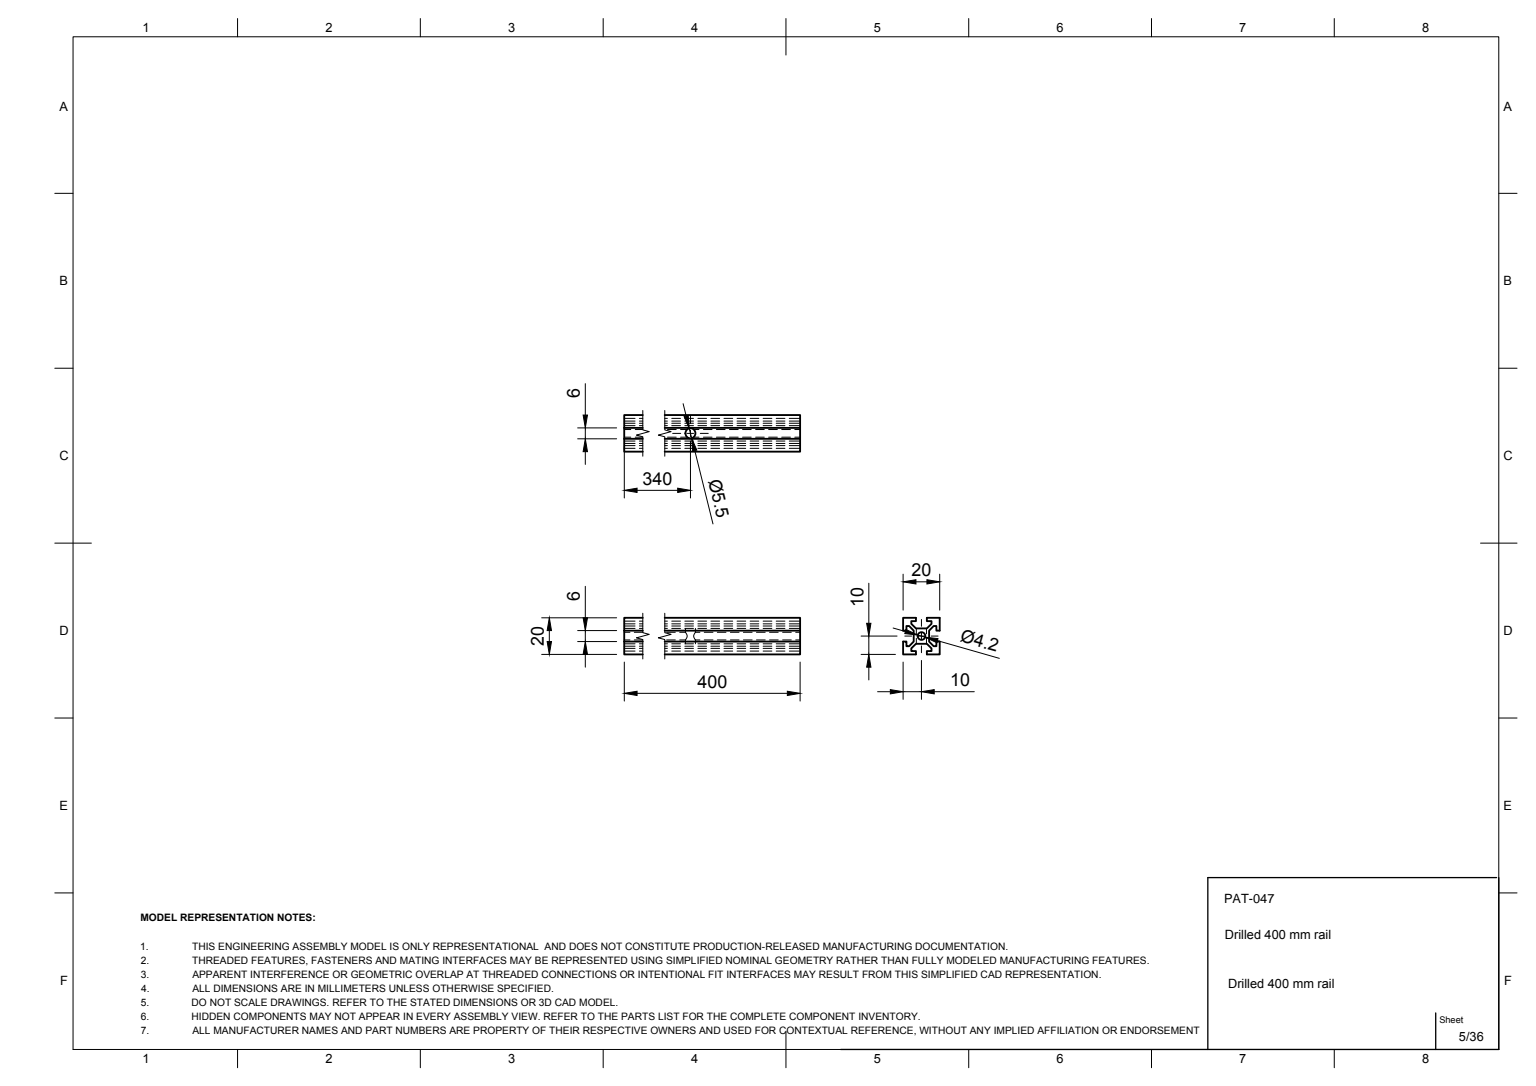
ISO-10303-21;
HEADER;
/* Generated by software containing ST-Developer
 * from STEP Tools, Inc. (www.steptools.com) 
 */

FILE_DESCRIPTION(
/* description */ ('Gravity roller conveyor section'),
/* implementation_level */ '2;1');

FILE_NAME(
/* name */ 'Drilled 400 mm rail.step',
/* time_stamp */ '2026-11-02T07:43:02-08:00',
/* author */ (''),
/* organization */ (''),
/* preprocessor_version */ 'ST-DEVELOPER v20.2',
/* originating_system */ 'Autodesk Translation Framework v15.17.0.0',
/* authorisation */ '');

FILE_SCHEMA (('AUTOMOTIVE_DESIGN { 1 0 10303 214 3 1 1 }'));
ENDSEC;

DATA;
#10=MECHANICAL_DESIGN_GEOMETRIC_PRESENTATION_REPRESENTATION('',(#530),#13821);
#433=B_SPLINE_CURVE_WITH_KNOTS('',3,(#11133,#11134,#11135,#11136,#11137,
#11138,#11139,#11140,#11141,#11142,#11143,#11144,#11145,#11146,#11147,#11148,
#11149,#11150,#11151,#11152,#11153,#11154),.UNSPECIFIED.,.F.,.F.,(4,2,2,
2,2,2,2,2,2,2,4),(0.335938049981194,0.418928967949028,0.501919885916861,
0.586897992939625,0.629387046451007,0.671876099962389,0.714365153473771,
0.756854206985153,0.841832314007917,0.92482323197575,1.00781414994358),
 .UNSPECIFIED.);
#434=B_SPLINE_CURVE_WITH_KNOTS('',3,(#11159,#11160,#11161,#11162,#11163,
#11164,#11165,#11166,#11167,#11168,#11169,#11170),.UNSPECIFIED.,.F.,.F.,
(4,2,2,2,2,4),(0.,0.0424890535113821,0.0849781070227642,0.169956214045528,
0.252947132013361,0.335938049981194),.UNSPECIFIED.);
#435=B_SPLINE_CURVE_WITH_KNOTS('',3,(#11171,#11172,#11173,#11174,#11175,
#11176,#11177,#11178,#11179,#11180,#11181,#11182),.UNSPECIFIED.,.F.,.F.,
(4,2,2,2,2,4),(1.00781414994358,1.09080506791142,1.17379598587925,1.25877409290201,
1.3012631464134,1.34375219992478),.UNSPECIFIED.);
#436=B_SPLINE_CURVE_WITH_KNOTS('',3,(#11185,#11186,#11187,#11188,#11189,
#11190,#11191,#11192,#11193,#11194,#11195,#11196,#11197,#11198,#11199,#11200,
#11201,#11202,#11203,#11204,#11205,#11206,#11207,#11208,#11209,#11210,#11211,
#11212,#11213,#11214,#11215,#11216),.UNSPECIFIED.,.F.,.F.,(4,2,2,2,2,2,
2,2,2,2,2,2,2,2,2,4),(0.,0.0424890535113822,0.0849781070227643,0.169956214045529,
0.252947132013362,0.335938049981195,0.418928967949028,0.501919885916861,
0.586897992939625,0.629387046451007,0.671876099962389,0.714365153473771,
0.756854206985153,0.841832314007917,0.924823231975751,1.00781414994358),
 .UNSPECIFIED.);
#437=B_SPLINE_CURVE_WITH_KNOTS('',3,(#11217,#11218,#11219,#11220,#11221,
#11222,#11223,#11224,#11225,#11226,#11227,#11228),.UNSPECIFIED.,.F.,.F.,
(4,2,2,2,2,4),(1.00781414994358,1.09080506791142,1.17379598587925,1.25877409290201,
1.3012631464134,1.34375219992478),.UNSPECIFIED.);
#462=SHAPE_REPRESENTATION_RELATIONSHIP('SRR','None',#13999,#496);
#496=ADVANCED_BREP_SHAPE_REPRESENTATION('',(#572),#13786);
#530=STYLED_ITEM('',(#14191),#572);
#572=MANIFOLD_SOLID_BREP('Body1',#7628);
#617=FACE_BOUND('',#1445,.T.);
#618=FACE_BOUND('',#1461,.T.);
#619=FACE_BOUND('',#1480,.T.);
#620=FACE_BOUND('',#1495,.T.);
#621=FACE_BOUND('',#1497,.T.);
#708=PLANE('',#8075);
#709=PLANE('',#8076);
#710=PLANE('',#8077);
#711=PLANE('',#8078);
#712=PLANE('',#8079);
#713=PLANE('',#8080);
#714=PLANE('',#8081);
#715=PLANE('',#8082);
#716=PLANE('',#8083);
#717=PLANE('',#8084);
#718=PLANE('',#8085);
#719=PLANE('',#8086);
#720=PLANE('',#8087);
#721=PLANE('',#8088);
#722=PLANE('',#8089);
#723=PLANE('',#8090);
#724=PLANE('',#8091);
#725=PLANE('',#8092);
#726=PLANE('',#8093);
#727=PLANE('',#8094);
#728=PLANE('',#8095);
#729=PLANE('',#8096);
#730=PLANE('',#8097);
#731=PLANE('',#8098);
#732=PLANE('',#8099);
#733=PLANE('',#8100);
#734=PLANE('',#8101);
#735=PLANE('',#8102);
#736=PLANE('',#8103);
#737=PLANE('',#8104);
#738=PLANE('',#8105);
#739=PLANE('',#8106);
#740=PLANE('',#8107);
#741=PLANE('',#8108);
#742=PLANE('',#8109);
#743=PLANE('',#8110);
#744=PLANE('',#8113);
#745=PLANE('',#8114);
#746=PLANE('',#8115);
#747=PLANE('',#8116);
#748=PLANE('',#8117);
#749=PLANE('',#8118);
#750=PLANE('',#8119);
#751=PLANE('',#8120);
#752=PLANE('',#8121);
#753=PLANE('',#8122);
#1017=FACE_OUTER_BOUND('',#1444,.T.);
#1018=FACE_OUTER_BOUND('',#1446,.T.);
#1019=FACE_OUTER_BOUND('',#1447,.T.);
#1020=FACE_OUTER_BOUND('',#1448,.T.);
#1021=FACE_OUTER_BOUND('',#1449,.T.);
#1022=FACE_OUTER_BOUND('',#1450,.T.);
#1023=FACE_OUTER_BOUND('',#1451,.T.);
#1024=FACE_OUTER_BOUND('',#1452,.T.);
#1025=FACE_OUTER_BOUND('',#1453,.T.);
#1026=FACE_OUTER_BOUND('',#1454,.T.);
#1027=FACE_OUTER_BOUND('',#1455,.T.);
#1028=FACE_OUTER_BOUND('',#1456,.T.);
#1029=FACE_OUTER_BOUND('',#1457,.T.);
#1030=FACE_OUTER_BOUND('',#1458,.T.);
#1031=FACE_OUTER_BOUND('',#1459,.T.);
#1032=FACE_OUTER_BOUND('',#1460,.T.);
#1033=FACE_OUTER_BOUND('',#1462,.T.);
#1034=FACE_OUTER_BOUND('',#1463,.T.);
#1035=FACE_OUTER_BOUND('',#1464,.T.);
#1036=FACE_OUTER_BOUND('',#1465,.T.);
#1037=FACE_OUTER_BOUND('',#1466,.T.);
#1038=FACE_OUTER_BOUND('',#1467,.T.);
#1039=FACE_OUTER_BOUND('',#1468,.T.);
#1040=FACE_OUTER_BOUND('',#1469,.T.);
#1041=FACE_OUTER_BOUND('',#1470,.T.);
#1042=FACE_OUTER_BOUND('',#1471,.T.);
#1043=FACE_OUTER_BOUND('',#1472,.T.);
#1044=FACE_OUTER_BOUND('',#1473,.T.);
#1045=FACE_OUTER_BOUND('',#1474,.T.);
#1046=FACE_OUTER_BOUND('',#1475,.T.);
#1047=FACE_OUTER_BOUND('',#1476,.T.);
#1048=FACE_OUTER_BOUND('',#1477,.T.);
#1049=FACE_OUTER_BOUND('',#1478,.T.);
#1050=FACE_OUTER_BOUND('',#1479,.T.);
#1051=FACE_OUTER_BOUND('',#1481,.T.);
#1052=FACE_OUTER_BOUND('',#1482,.T.);
#1053=FACE_OUTER_BOUND('',#1483,.T.);
#1054=FACE_OUTER_BOUND('',#1484,.T.);
#1055=FACE_OUTER_BOUND('',#1485,.T.);
#1056=FACE_OUTER_BOUND('',#1486,.T.);
#1057=FACE_OUTER_BOUND('',#1487,.T.);
#1058=FACE_OUTER_BOUND('',#1488,.T.);
#1059=FACE_OUTER_BOUND('',#1489,.T.);
#1060=FACE_OUTER_BOUND('',#1490,.T.);
#1061=FACE_OUTER_BOUND('',#1491,.T.);
#1062=FACE_OUTER_BOUND('',#1492,.T.);
#1063=FACE_OUTER_BOUND('',#1493,.T.);
#1064=FACE_OUTER_BOUND('',#1494,.T.);
#1065=FACE_OUTER_BOUND('',#1496,.T.);
#1444=EDGE_LOOP('',(#5250,#5251,#5252,#5253,#5254,#5255,#5256,#5257,#5258));
#1445=EDGE_LOOP('',(#5259,#5260));
#1446=EDGE_LOOP('',(#5261,#5262,#5263,#5264,#5265,#5266));
#1447=EDGE_LOOP('',(#5267,#5268,#5269,#5270));
#1448=EDGE_LOOP('',(#5271,#5272,#5273,#5274));
#1449=EDGE_LOOP('',(#5275,#5276,#5277,#5278));
#1450=EDGE_LOOP('',(#5279,#5280,#5281,#5282));
#1451=EDGE_LOOP('',(#5283,#5284,#5285,#5286));
#1452=EDGE_LOOP('',(#5287,#5288,#5289,#5290));
#1453=EDGE_LOOP('',(#5291,#5292,#5293,#5294));
#1454=EDGE_LOOP('',(#5295,#5296,#5297,#5298));
#1455=EDGE_LOOP('',(#5299,#5300,#5301,#5302));
#1456=EDGE_LOOP('',(#5303,#5304,#5305,#5306));
#1457=EDGE_LOOP('',(#5307,#5308,#5309,#5310));
#1458=EDGE_LOOP('',(#5311,#5312,#5313,#5314));
#1459=EDGE_LOOP('',(#5315,#5316,#5317,#5318));
#1460=EDGE_LOOP('',(#5319,#5320,#5321,#5322));
#1461=EDGE_LOOP('',(#5323));
#1462=EDGE_LOOP('',(#5324,#5325,#5326,#5327));
#1463=EDGE_LOOP('',(#5328,#5329,#5330,#5331));
#1464=EDGE_LOOP('',(#5332,#5333,#5334,#5335));
#1465=EDGE_LOOP('',(#5336,#5337,#5338,#5339));
#1466=EDGE_LOOP('',(#5340,#5341,#5342,#5343));
#1467=EDGE_LOOP('',(#5344,#5345,#5346,#5347));
#1468=EDGE_LOOP('',(#5348,#5349,#5350,#5351));
#1469=EDGE_LOOP('',(#5352,#5353,#5354,#5355));
#1470=EDGE_LOOP('',(#5356,#5357,#5358,#5359));
#1471=EDGE_LOOP('',(#5360,#5361,#5362,#5363));
#1472=EDGE_LOOP('',(#5364,#5365,#5366,#5367));
#1473=EDGE_LOOP('',(#5368,#5369,#5370,#5371));
#1474=EDGE_LOOP('',(#5372,#5373,#5374,#5375));
#1475=EDGE_LOOP('',(#5376,#5377,#5378,#5379));
#1476=EDGE_LOOP('',(#5380,#5381,#5382,#5383));
#1477=EDGE_LOOP('',(#5384,#5385,#5386,#5387));
#1478=EDGE_LOOP('',(#5388,#5389,#5390,#5391));
#1479=EDGE_LOOP('',(#5392,#5393,#5394,#5395));
#1480=EDGE_LOOP('',(#5396));
#1481=EDGE_LOOP('',(#5397,#5398,#5399,#5400));
#1482=EDGE_LOOP('',(#5401,#5402,#5403,#5404));
#1483=EDGE_LOOP('',(#5405,#5406,#5407,#5408));
#1484=EDGE_LOOP('',(#5409,#5410,#5411,#5412));
#1485=EDGE_LOOP('',(#5413,#5414,#5415,#5416,#5417));
#1486=EDGE_LOOP('',(#5418,#5419,#5420,#5421));
#1487=EDGE_LOOP('',(#5422,#5423,#5424,#5425));
#1488=EDGE_LOOP('',(#5426,#5427,#5428,#5429));
#1489=EDGE_LOOP('',(#5430,#5431,#5432,#5433));
#1490=EDGE_LOOP('',(#5434,#5435,#5436,#5437));
#1491=EDGE_LOOP('',(#5438,#5439,#5440,#5441));
#1492=EDGE_LOOP('',(#5442,#5443,#5444,#5445));
#1493=EDGE_LOOP('',(#5446,#5447,#5448,#5449));
#1494=EDGE_LOOP('',(#5450,#5451,#5452,#5453,#5454,#5455,#5456,#5457,#5458,
#5459,#5460,#5461,#5462,#5463,#5464,#5465,#5466,#5467,#5468,#5469,#5470,
#5471,#5472,#5473,#5474,#5475,#5476,#5477,#5478,#5479,#5480,#5481,#5482,
#5483,#5484,#5485,#5486,#5487,#5488,#5489,#5490,#5491,#5492,#5493));
#1495=EDGE_LOOP('',(#5494));
#1496=EDGE_LOOP('',(#5495,#5496,#5497,#5498,#5499,#5500,#5501,#5502,#5503,
#5504,#5505,#5506,#5507,#5508,#5509,#5510,#5511,#5512,#5513,#5514,#5515,
#5516,#5517,#5518,#5519,#5520,#5521,#5522,#5523,#5524,#5525,#5526,#5527,
#5528,#5529,#5530,#5531,#5532,#5533,#5534,#5535,#5536,#5537,#5538));
#1497=EDGE_LOOP('',(#5539));
#1954=LINE('',#11131,#2672);
#1955=LINE('',#11156,#2673);
#1956=LINE('',#11232,#2674);
#1957=LINE('',#11236,#2675);
#1958=LINE('',#11238,#2676);
#1959=LINE('',#11240,#2677);
#1960=LINE('',#11241,#2678);
#1961=LINE('',#11244,#2679);
#1962=LINE('',#11246,#2680);
#1963=LINE('',#11247,#2681);
#1964=LINE('',#11250,#2682);
#1965=LINE('',#11252,#2683);
#1966=LINE('',#11253,#2684);
#1967=LINE('',#11256,#2685);
#1968=LINE('',#11258,#2686);
#1969=LINE('',#11259,#2687);
#1970=LINE('',#11262,#2688);
#1971=LINE('',#11264,#2689);
#1972=LINE('',#11265,#2690);
#1973=LINE('',#11268,#2691);
#1974=LINE('',#11270,#2692);
#1975=LINE('',#11271,#2693);
#1976=LINE('',#11274,#2694);
#1977=LINE('',#11276,#2695);
#1978=LINE('',#11277,#2696);
#1979=LINE('',#11280,#2697);
#1980=LINE('',#11282,#2698);
#1981=LINE('',#11283,#2699);
#1982=LINE('',#11286,#2700);
#1983=LINE('',#11288,#2701);
#1984=LINE('',#11289,#2702);
#1985=LINE('',#11293,#2703);
#1986=LINE('',#11295,#2704);
#1987=LINE('',#11297,#2705);
#1988=LINE('',#11298,#2706);
#1989=LINE('',#11301,#2707);
#1990=LINE('',#11303,#2708);
#1991=LINE('',#11304,#2709);
#1992=LINE('',#11307,#2710);
#1993=LINE('',#11309,#2711);
#1994=LINE('',#11310,#2712);
#1995=LINE('',#11313,#2713);
#1996=LINE('',#11315,#2714);
#1997=LINE('',#11316,#2715);
#1998=LINE('',#11319,#2716);
#1999=LINE('',#11321,#2717);
#2000=LINE('',#11322,#2718);
#2001=LINE('',#11325,#2719);
#2002=LINE('',#11327,#2720);
#2003=LINE('',#11328,#2721);
#2004=LINE('',#11331,#2722);
#2005=LINE('',#11333,#2723);
#2006=LINE('',#11334,#2724);
#2007=LINE('',#11337,#2725);
#2008=LINE('',#11339,#2726);
#2009=LINE('',#11340,#2727);
#2010=LINE('',#11343,#2728);
#2011=LINE('',#11345,#2729);
#2012=LINE('',#11346,#2730);
#2013=LINE('',#11350,#2731);
#2014=LINE('',#11352,#2732);
#2015=LINE('',#11354,#2733);
#2016=LINE('',#11355,#2734);
#2017=LINE('',#11358,#2735);
#2018=LINE('',#11360,#2736);
#2019=LINE('',#11361,#2737);
#2020=LINE('',#11364,#2738);
#2021=LINE('',#11366,#2739);
#2022=LINE('',#11367,#2740);
#2023=LINE('',#11370,#2741);
#2024=LINE('',#11372,#2742);
#2025=LINE('',#11373,#2743);
#2026=LINE('',#11376,#2744);
#2027=LINE('',#11378,#2745);
#2028=LINE('',#11379,#2746);
#2029=LINE('',#11382,#2747);
#2030=LINE('',#11384,#2748);
#2031=LINE('',#11385,#2749);
#2032=LINE('',#11388,#2750);
#2033=LINE('',#11390,#2751);
#2034=LINE('',#11391,#2752);
#2035=LINE('',#11394,#2753);
#2036=LINE('',#11396,#2754);
#2037=LINE('',#11397,#2755);
#2038=LINE('',#11400,#2756);
#2039=LINE('',#11402,#2757);
#2040=LINE('',#11403,#2758);
#2041=LINE('',#11407,#2759);
#2042=LINE('',#11409,#2760);
#2043=LINE('',#11411,#2761);
#2044=LINE('',#11412,#2762);
#2045=LINE('',#11415,#2763);
#2046=LINE('',#11417,#2764);
#2047=LINE('',#11418,#2765);
#2048=LINE('',#11421,#2766);
#2049=LINE('',#11423,#2767);
#2050=LINE('',#11424,#2768);
#2051=LINE('',#11427,#2769);
#2052=LINE('',#11429,#2770);
#2053=LINE('',#11430,#2771);
#2054=LINE('',#11433,#2772);
#2055=LINE('',#11435,#2773);
#2056=LINE('',#11436,#2774);
#2057=LINE('',#11439,#2775);
#2058=LINE('',#11441,#2776);
#2059=LINE('',#11442,#2777);
#2060=LINE('',#11445,#2778);
#2061=LINE('',#11447,#2779);
#2062=LINE('',#11448,#2780);
#2063=LINE('',#11451,#2781);
#2064=LINE('',#11453,#2782);
#2065=LINE('',#11454,#2783);
#2066=LINE('',#11457,#2784);
#2067=LINE('',#11459,#2785);
#2068=LINE('',#11460,#2786);
#2069=LINE('',#11463,#2787);
#2070=LINE('',#11467,#2788);
#2071=LINE('',#11469,#2789);
#2072=LINE('',#11470,#2790);
#2073=LINE('',#11473,#2791);
#2074=LINE('',#11475,#2792);
#2075=LINE('',#11476,#2793);
#2076=LINE('',#11478,#2794);
#2077=LINE('',#11479,#2795);
#2078=LINE('',#11482,#2796);
#2079=LINE('',#11484,#2797);
#2080=LINE('',#11485,#2798);
#2081=LINE('',#11487,#2799);
#2082=LINE('',#11488,#2800);
#2083=LINE('',#11491,#2801);
#2084=LINE('',#11493,#2802);
#2085=LINE('',#11494,#2803);
#2086=LINE('',#11496,#2804);
#2087=LINE('',#11497,#2805);
#2088=LINE('',#11499,#2806);
#2089=LINE('',#11500,#2807);
#2672=VECTOR('',#8881,0.275);
#2673=VECTOR('',#8882,0.275);
#2674=VECTOR('',#8889,0.21);
#2675=VECTOR('',#8892,1.);
#2676=VECTOR('',#8893,1.);
#2677=VECTOR('',#8894,1.);
#2678=VECTOR('',#8895,1.);
#2679=VECTOR('',#8898,1.);
#2680=VECTOR('',#8899,1.);
#2681=VECTOR('',#8900,1.);
#2682=VECTOR('',#8903,1.);
#2683=VECTOR('',#8904,1.);
#2684=VECTOR('',#8905,1.);
#2685=VECTOR('',#8908,1.);
#2686=VECTOR('',#8909,1.);
#2687=VECTOR('',#8910,1.);
#2688=VECTOR('',#8913,1.);
#2689=VECTOR('',#8914,1.);
#2690=VECTOR('',#8915,1.);
#2691=VECTOR('',#8918,1.);
#2692=VECTOR('',#8919,1.);
#2693=VECTOR('',#8920,1.);
#2694=VECTOR('',#8923,1.);
#2695=VECTOR('',#8924,1.);
#2696=VECTOR('',#8925,1.);
#2697=VECTOR('',#8928,1.);
#2698=VECTOR('',#8929,1.);
#2699=VECTOR('',#8930,1.);
#2700=VECTOR('',#8933,1.);
#2701=VECTOR('',#8934,1.);
#2702=VECTOR('',#8935,1.);
#2703=VECTOR('',#8938,1.);
#2704=VECTOR('',#8939,1.);
#2705=VECTOR('',#8940,1.);
#2706=VECTOR('',#8941,1.);
#2707=VECTOR('',#8944,1.);
#2708=VECTOR('',#8945,1.);
#2709=VECTOR('',#8946,1.);
#2710=VECTOR('',#8949,1.);
#2711=VECTOR('',#8950,1.);
#2712=VECTOR('',#8951,1.);
#2713=VECTOR('',#8954,1.);
#2714=VECTOR('',#8955,1.);
#2715=VECTOR('',#8956,1.);
#2716=VECTOR('',#8959,1.);
#2717=VECTOR('',#8960,1.);
#2718=VECTOR('',#8961,1.);
#2719=VECTOR('',#8964,1.);
#2720=VECTOR('',#8965,1.);
#2721=VECTOR('',#8966,1.);
#2722=VECTOR('',#8969,1.);
#2723=VECTOR('',#8970,1.);
#2724=VECTOR('',#8971,1.);
#2725=VECTOR('',#8974,1.);
#2726=VECTOR('',#8975,1.);
#2727=VECTOR('',#8976,1.);
#2728=VECTOR('',#8979,1.);
#2729=VECTOR('',#8980,1.);
#2730=VECTOR('',#8981,1.);
#2731=VECTOR('',#8984,1.);
#2732=VECTOR('',#8985,1.);
#2733=VECTOR('',#8986,1.);
#2734=VECTOR('',#8987,1.);
#2735=VECTOR('',#8990,1.);
#2736=VECTOR('',#8991,1.);
#2737=VECTOR('',#8992,1.);
#2738=VECTOR('',#8995,1.);
#2739=VECTOR('',#8996,1.);
#2740=VECTOR('',#8997,1.);
#2741=VECTOR('',#9000,1.);
#2742=VECTOR('',#9001,1.);
#2743=VECTOR('',#9002,1.);
#2744=VECTOR('',#9005,1.);
#2745=VECTOR('',#9006,1.);
#2746=VECTOR('',#9007,1.);
#2747=VECTOR('',#9010,1.);
#2748=VECTOR('',#9011,1.);
#2749=VECTOR('',#9012,1.);
#2750=VECTOR('',#9015,1.);
#2751=VECTOR('',#9016,1.);
#2752=VECTOR('',#9017,1.);
#2753=VECTOR('',#9020,1.);
#2754=VECTOR('',#9021,1.);
#2755=VECTOR('',#9022,1.);
#2756=VECTOR('',#9025,1.);
#2757=VECTOR('',#9026,1.);
#2758=VECTOR('',#9027,1.);
#2759=VECTOR('',#9030,1.);
#2760=VECTOR('',#9031,1.);
#2761=VECTOR('',#9032,1.);
#2762=VECTOR('',#9033,1.);
#2763=VECTOR('',#9036,1.);
#2764=VECTOR('',#9037,1.);
#2765=VECTOR('',#9038,1.);
#2766=VECTOR('',#9041,1.);
#2767=VECTOR('',#9042,1.);
#2768=VECTOR('',#9043,1.);
#2769=VECTOR('',#9046,1.);
#2770=VECTOR('',#9047,1.);
#2771=VECTOR('',#9048,1.);
#2772=VECTOR('',#9051,1.);
#2773=VECTOR('',#9052,1.);
#2774=VECTOR('',#9053,1.);
#2775=VECTOR('',#9056,1.);
#2776=VECTOR('',#9057,1.);
#2777=VECTOR('',#9058,1.);
#2778=VECTOR('',#9061,1.);
#2779=VECTOR('',#9062,1.);
#2780=VECTOR('',#9063,1.);
#2781=VECTOR('',#9066,1.);
#2782=VECTOR('',#9067,1.);
#2783=VECTOR('',#9068,1.);
#2784=VECTOR('',#9071,1.);
#2785=VECTOR('',#9072,1.);
#2786=VECTOR('',#9073,1.);
#2787=VECTOR('',#9076,0.21);
#2788=VECTOR('',#9081,1.);
#2789=VECTOR('',#9082,1.);
#2790=VECTOR('',#9083,1.);
#2791=VECTOR('',#9086,1.);
#2792=VECTOR('',#9087,1.);
#2793=VECTOR('',#9088,1.);
#2794=VECTOR('',#9091,1.);
#2795=VECTOR('',#9092,1.);
#2796=VECTOR('',#9095,1.);
#2797=VECTOR('',#9096,1.);
#2798=VECTOR('',#9097,1.);
#2799=VECTOR('',#9100,1.);
#2800=VECTOR('',#9101,1.);
#2801=VECTOR('',#9104,1.);
#2802=VECTOR('',#9105,1.);
#2803=VECTOR('',#9106,1.);
#2804=VECTOR('',#9109,1.);
#2805=VECTOR('',#9110,1.);
#2806=VECTOR('',#9113,1.);
#2807=VECTOR('',#9114,1.);
#3382=CIRCLE('',#8071,0.275);
#3383=CIRCLE('',#8072,0.275);
#3384=CIRCLE('',#8074,0.21);
#3385=CIRCLE('',#8112,0.21);
#3606=VERTEX_POINT('',#11128);
#3607=VERTEX_POINT('',#11130);
#3608=VERTEX_POINT('',#11132);
#3609=VERTEX_POINT('',#11155);
#3610=VERTEX_POINT('',#11158);
#3611=VERTEX_POINT('',#11183);
#3612=VERTEX_POINT('',#11184);
#3613=VERTEX_POINT('',#11230);
#3614=VERTEX_POINT('',#11234);
#3615=VERTEX_POINT('',#11235);
#3616=VERTEX_POINT('',#11237);
#3617=VERTEX_POINT('',#11239);
#3618=VERTEX_POINT('',#11243);
#3619=VERTEX_POINT('',#11245);
#3620=VERTEX_POINT('',#11249);
#3621=VERTEX_POINT('',#11251);
#3622=VERTEX_POINT('',#11255);
#3623=VERTEX_POINT('',#11257);
#3624=VERTEX_POINT('',#11261);
#3625=VERTEX_POINT('',#11263);
#3626=VERTEX_POINT('',#11267);
#3627=VERTEX_POINT('',#11269);
#3628=VERTEX_POINT('',#11273);
#3629=VERTEX_POINT('',#11275);
#3630=VERTEX_POINT('',#11279);
#3631=VERTEX_POINT('',#11281);
#3632=VERTEX_POINT('',#11285);
#3633=VERTEX_POINT('',#11287);
#3634=VERTEX_POINT('',#11291);
#3635=VERTEX_POINT('',#11292);
#3636=VERTEX_POINT('',#11294);
#3637=VERTEX_POINT('',#11296);
#3638=VERTEX_POINT('',#11300);
#3639=VERTEX_POINT('',#11302);
#3640=VERTEX_POINT('',#11306);
#3641=VERTEX_POINT('',#11308);
#3642=VERTEX_POINT('',#11312);
#3643=VERTEX_POINT('',#11314);
#3644=VERTEX_POINT('',#11318);
#3645=VERTEX_POINT('',#11320);
#3646=VERTEX_POINT('',#11324);
#3647=VERTEX_POINT('',#11326);
#3648=VERTEX_POINT('',#11330);
#3649=VERTEX_POINT('',#11332);
#3650=VERTEX_POINT('',#11336);
#3651=VERTEX_POINT('',#11338);
#3652=VERTEX_POINT('',#11342);
#3653=VERTEX_POINT('',#11344);
#3654=VERTEX_POINT('',#11348);
#3655=VERTEX_POINT('',#11349);
#3656=VERTEX_POINT('',#11351);
#3657=VERTEX_POINT('',#11353);
#3658=VERTEX_POINT('',#11357);
#3659=VERTEX_POINT('',#11359);
#3660=VERTEX_POINT('',#11363);
#3661=VERTEX_POINT('',#11365);
#3662=VERTEX_POINT('',#11369);
#3663=VERTEX_POINT('',#11371);
#3664=VERTEX_POINT('',#11375);
#3665=VERTEX_POINT('',#11377);
#3666=VERTEX_POINT('',#11381);
#3667=VERTEX_POINT('',#11383);
#3668=VERTEX_POINT('',#11387);
#3669=VERTEX_POINT('',#11389);
#3670=VERTEX_POINT('',#11393);
#3671=VERTEX_POINT('',#11395);
#3672=VERTEX_POINT('',#11399);
#3673=VERTEX_POINT('',#11401);
#3674=VERTEX_POINT('',#11405);
#3675=VERTEX_POINT('',#11406);
#3676=VERTEX_POINT('',#11408);
#3677=VERTEX_POINT('',#11410);
#3678=VERTEX_POINT('',#11414);
#3679=VERTEX_POINT('',#11416);
#3680=VERTEX_POINT('',#11420);
#3681=VERTEX_POINT('',#11422);
#3682=VERTEX_POINT('',#11426);
#3683=VERTEX_POINT('',#11428);
#3684=VERTEX_POINT('',#11432);
#3685=VERTEX_POINT('',#11434);
#3686=VERTEX_POINT('',#11438);
#3687=VERTEX_POINT('',#11440);
#3688=VERTEX_POINT('',#11444);
#3689=VERTEX_POINT('',#11446);
#3690=VERTEX_POINT('',#11450);
#3691=VERTEX_POINT('',#11452);
#3692=VERTEX_POINT('',#11456);
#3693=VERTEX_POINT('',#11458);
#3694=VERTEX_POINT('',#11462);
#3695=VERTEX_POINT('',#11466);
#3696=VERTEX_POINT('',#11468);
#3697=VERTEX_POINT('',#11472);
#3698=VERTEX_POINT('',#11474);
#3699=VERTEX_POINT('',#11481);
#3700=VERTEX_POINT('',#11483);
#3701=VERTEX_POINT('',#11490);
#3702=VERTEX_POINT('',#11492);
#4262=EDGE_CURVE('',#3606,#3606,#3382,.T.);
#4263=EDGE_CURVE('',#3606,#3607,#1954,.T.);
#4264=EDGE_CURVE('',#3608,#3607,#433,.T.);
#4265=EDGE_CURVE('',#3608,#3609,#1955,.T.);
#4266=EDGE_CURVE('',#3609,#3609,#3383,.T.);
#4267=EDGE_CURVE('',#3610,#3608,#434,.T.);
#4268=EDGE_CURVE('',#3607,#3610,#435,.T.);
#4269=EDGE_CURVE('',#3611,#3612,#436,.T.);
#4270=EDGE_CURVE('',#3612,#3611,#437,.T.);
#4271=EDGE_CURVE('',#3613,#3613,#3384,.T.);
#4272=EDGE_CURVE('',#3613,#3608,#1956,.T.);
#4273=EDGE_CURVE('',#3614,#3615,#1957,.T.);
#4274=EDGE_CURVE('',#3614,#3616,#1958,.T.);
#4275=EDGE_CURVE('',#3617,#3616,#1959,.T.);
#4276=EDGE_CURVE('',#3615,#3617,#1960,.T.);
#4277=EDGE_CURVE('',#3618,#3614,#1961,.T.);
#4278=EDGE_CURVE('',#3618,#3619,#1962,.T.);
#4279=EDGE_CURVE('',#3616,#3619,#1963,.T.);
#4280=EDGE_CURVE('',#3620,#3618,#1964,.T.);
#4281=EDGE_CURVE('',#3620,#3621,#1965,.T.);
#4282=EDGE_CURVE('',#3619,#3621,#1966,.T.);
#4283=EDGE_CURVE('',#3622,#3620,#1967,.T.);
#4284=EDGE_CURVE('',#3622,#3623,#1968,.T.);
#4285=EDGE_CURVE('',#3621,#3623,#1969,.T.);
#4286=EDGE_CURVE('',#3624,#3622,#1970,.T.);
#4287=EDGE_CURVE('',#3624,#3625,#1971,.T.);
#4288=EDGE_CURVE('',#3623,#3625,#1972,.T.);
#4289=EDGE_CURVE('',#3626,#3624,#1973,.T.);
#4290=EDGE_CURVE('',#3626,#3627,#1974,.T.);
#4291=EDGE_CURVE('',#3625,#3627,#1975,.T.);
#4292=EDGE_CURVE('',#3628,#3626,#1976,.T.);
#4293=EDGE_CURVE('',#3628,#3629,#1977,.T.);
#4294=EDGE_CURVE('',#3627,#3629,#1978,.T.);
#4295=EDGE_CURVE('',#3630,#3628,#1979,.T.);
#4296=EDGE_CURVE('',#3630,#3631,#1980,.T.);
#4297=EDGE_CURVE('',#3629,#3631,#1981,.T.);
#4298=EDGE_CURVE('',#3632,#3630,#1982,.T.);
#4299=EDGE_CURVE('',#3633,#3632,#1983,.T.);
#4300=EDGE_CURVE('',#3631,#3633,#1984,.T.);
#4301=EDGE_CURVE('',#3634,#3635,#1985,.T.);
#4302=EDGE_CURVE('',#3634,#3636,#1986,.T.);
#4303=EDGE_CURVE('',#3637,#3636,#1987,.T.);
#4304=EDGE_CURVE('',#3635,#3637,#1988,.T.);
#4305=EDGE_CURVE('',#3638,#3634,#1989,.T.);
#4306=EDGE_CURVE('',#3638,#3639,#1990,.T.);
#4307=EDGE_CURVE('',#3636,#3639,#1991,.T.);
#4308=EDGE_CURVE('',#3640,#3638,#1992,.T.);
#4309=EDGE_CURVE('',#3640,#3641,#1993,.T.);
#4310=EDGE_CURVE('',#3639,#3641,#1994,.T.);
#4311=EDGE_CURVE('',#3642,#3640,#1995,.T.);
#4312=EDGE_CURVE('',#3642,#3643,#1996,.T.);
#4313=EDGE_CURVE('',#3641,#3643,#1997,.T.);
#4314=EDGE_CURVE('',#3644,#3642,#1998,.T.);
#4315=EDGE_CURVE('',#3644,#3645,#1999,.T.);
#4316=EDGE_CURVE('',#3643,#3645,#2000,.T.);
#4317=EDGE_CURVE('',#3646,#3644,#2001,.T.);
#4318=EDGE_CURVE('',#3646,#3647,#2002,.T.);
#4319=EDGE_CURVE('',#3645,#3647,#2003,.T.);
#4320=EDGE_CURVE('',#3648,#3646,#2004,.T.);
#4321=EDGE_CURVE('',#3648,#3649,#2005,.T.);
#4322=EDGE_CURVE('',#3647,#3649,#2006,.T.);
#4323=EDGE_CURVE('',#3650,#3648,#2007,.T.);
#4324=EDGE_CURVE('',#3650,#3651,#2008,.T.);
#4325=EDGE_CURVE('',#3649,#3651,#2009,.T.);
#4326=EDGE_CURVE('',#3652,#3650,#2010,.T.);
#4327=EDGE_CURVE('',#3653,#3652,#2011,.T.);
#4328=EDGE_CURVE('',#3651,#3653,#2012,.T.);
#4329=EDGE_CURVE('',#3654,#3655,#2013,.T.);
#4330=EDGE_CURVE('',#3654,#3656,#2014,.T.);
#4331=EDGE_CURVE('',#3657,#3656,#2015,.T.);
#4332=EDGE_CURVE('',#3655,#3657,#2016,.T.);
#4333=EDGE_CURVE('',#3658,#3654,#2017,.T.);
#4334=EDGE_CURVE('',#3658,#3659,#2018,.T.);
#4335=EDGE_CURVE('',#3656,#3659,#2019,.T.);
#4336=EDGE_CURVE('',#3660,#3658,#2020,.T.);
#4337=EDGE_CURVE('',#3660,#3661,#2021,.T.);
#4338=EDGE_CURVE('',#3659,#3661,#2022,.T.);
#4339=EDGE_CURVE('',#3662,#3660,#2023,.T.);
#4340=EDGE_CURVE('',#3662,#3663,#2024,.T.);
#4341=EDGE_CURVE('',#3661,#3663,#2025,.T.);
#4342=EDGE_CURVE('',#3664,#3662,#2026,.T.);
#4343=EDGE_CURVE('',#3664,#3665,#2027,.T.);
#4344=EDGE_CURVE('',#3663,#3665,#2028,.T.);
#4345=EDGE_CURVE('',#3666,#3664,#2029,.T.);
#4346=EDGE_CURVE('',#3666,#3667,#2030,.T.);
#4347=EDGE_CURVE('',#3665,#3667,#2031,.T.);
#4348=EDGE_CURVE('',#3668,#3666,#2032,.T.);
#4349=EDGE_CURVE('',#3668,#3669,#2033,.T.);
#4350=EDGE_CURVE('',#3667,#3669,#2034,.T.);
#4351=EDGE_CURVE('',#3670,#3668,#2035,.T.);
#4352=EDGE_CURVE('',#3670,#3671,#2036,.T.);
#4353=EDGE_CURVE('',#3669,#3671,#2037,.T.);
#4354=EDGE_CURVE('',#3672,#3670,#2038,.T.);
#4355=EDGE_CURVE('',#3673,#3672,#2039,.T.);
#4356=EDGE_CURVE('',#3671,#3673,#2040,.T.);
#4357=EDGE_CURVE('',#3674,#3675,#2041,.T.);
#4358=EDGE_CURVE('',#3674,#3676,#2042,.T.);
#4359=EDGE_CURVE('',#3677,#3676,#2043,.T.);
#4360=EDGE_CURVE('',#3675,#3677,#2044,.T.);
#4361=EDGE_CURVE('',#3678,#3674,#2045,.T.);
#4362=EDGE_CURVE('',#3678,#3679,#2046,.T.);
#4363=EDGE_CURVE('',#3676,#3679,#2047,.T.);
#4364=EDGE_CURVE('',#3680,#3678,#2048,.T.);
#4365=EDGE_CURVE('',#3680,#3681,#2049,.T.);
#4366=EDGE_CURVE('',#3679,#3681,#2050,.T.);
#4367=EDGE_CURVE('',#3682,#3680,#2051,.T.);
#4368=EDGE_CURVE('',#3682,#3683,#2052,.T.);
#4369=EDGE_CURVE('',#3681,#3683,#2053,.T.);
#4370=EDGE_CURVE('',#3684,#3682,#2054,.T.);
#4371=EDGE_CURVE('',#3684,#3685,#2055,.T.);
#4372=EDGE_CURVE('',#3683,#3685,#2056,.T.);
#4373=EDGE_CURVE('',#3686,#3684,#2057,.T.);
#4374=EDGE_CURVE('',#3686,#3687,#2058,.T.);
#4375=EDGE_CURVE('',#3685,#3687,#2059,.T.);
#4376=EDGE_CURVE('',#3688,#3686,#2060,.T.);
#4377=EDGE_CURVE('',#3688,#3689,#2061,.T.);
#4378=EDGE_CURVE('',#3687,#3689,#2062,.T.);
#4379=EDGE_CURVE('',#3690,#3688,#2063,.T.);
#4380=EDGE_CURVE('',#3690,#3691,#2064,.T.);
#4381=EDGE_CURVE('',#3689,#3691,#2065,.T.);
#4382=EDGE_CURVE('',#3692,#3690,#2066,.T.);
#4383=EDGE_CURVE('',#3693,#3692,#2067,.T.);
#4384=EDGE_CURVE('',#3691,#3693,#2068,.T.);
#4385=EDGE_CURVE('',#3612,#3694,#2069,.T.);
#4386=EDGE_CURVE('',#3694,#3694,#3385,.T.);
#4387=EDGE_CURVE('',#3632,#3695,#2070,.T.);
#4388=EDGE_CURVE('',#3695,#3696,#2071,.T.);
#4389=EDGE_CURVE('',#3633,#3696,#2072,.T.);
#4390=EDGE_CURVE('',#3697,#3617,#2073,.T.);
#4391=EDGE_CURVE('',#3698,#3697,#2074,.T.);
#4392=EDGE_CURVE('',#3698,#3615,#2075,.T.);
#4393=EDGE_CURVE('',#3652,#3698,#2076,.T.);
#4394=EDGE_CURVE('',#3653,#3697,#2077,.T.);
#4395=EDGE_CURVE('',#3699,#3637,#2078,.T.);
#4396=EDGE_CURVE('',#3700,#3699,#2079,.T.);
#4397=EDGE_CURVE('',#3700,#3635,#2080,.T.);
#4398=EDGE_CURVE('',#3672,#3700,#2081,.T.);
#4399=EDGE_CURVE('',#3673,#3699,#2082,.T.);
#4400=EDGE_CURVE('',#3701,#3657,#2083,.T.);
#4401=EDGE_CURVE('',#3702,#3701,#2084,.T.);
#4402=EDGE_CURVE('',#3702,#3655,#2085,.T.);
#4403=EDGE_CURVE('',#3692,#3702,#2086,.T.);
#4404=EDGE_CURVE('',#3693,#3701,#2087,.T.);
#4405=EDGE_CURVE('',#3696,#3677,#2088,.T.);
#4406=EDGE_CURVE('',#3695,#3675,#2089,.T.);
#5250=ORIENTED_EDGE('',*,*,#4262,.F.);
#5251=ORIENTED_EDGE('',*,*,#4263,.T.);
#5252=ORIENTED_EDGE('',*,*,#4264,.F.);
#5253=ORIENTED_EDGE('',*,*,#4265,.T.);
#5254=ORIENTED_EDGE('',*,*,#4266,.F.);
#5255=ORIENTED_EDGE('',*,*,#4265,.F.);
#5256=ORIENTED_EDGE('',*,*,#4267,.F.);
#5257=ORIENTED_EDGE('',*,*,#4268,.F.);
#5258=ORIENTED_EDGE('',*,*,#4263,.F.);
#5259=ORIENTED_EDGE('',*,*,#4269,.F.);
#5260=ORIENTED_EDGE('',*,*,#4270,.F.);
#5261=ORIENTED_EDGE('',*,*,#4271,.F.);
#5262=ORIENTED_EDGE('',*,*,#4272,.T.);
#5263=ORIENTED_EDGE('',*,*,#4264,.T.);
#5264=ORIENTED_EDGE('',*,*,#4268,.T.);
#5265=ORIENTED_EDGE('',*,*,#4267,.T.);
#5266=ORIENTED_EDGE('',*,*,#4272,.F.);
#5267=ORIENTED_EDGE('',*,*,#4273,.F.);
#5268=ORIENTED_EDGE('',*,*,#4274,.T.);
#5269=ORIENTED_EDGE('',*,*,#4275,.F.);
#5270=ORIENTED_EDGE('',*,*,#4276,.F.);
#5271=ORIENTED_EDGE('',*,*,#4277,.F.);
#5272=ORIENTED_EDGE('',*,*,#4278,.T.);
#5273=ORIENTED_EDGE('',*,*,#4279,.F.);
#5274=ORIENTED_EDGE('',*,*,#4274,.F.);
#5275=ORIENTED_EDGE('',*,*,#4280,.F.);
#5276=ORIENTED_EDGE('',*,*,#4281,.T.);
#5277=ORIENTED_EDGE('',*,*,#4282,.F.);
#5278=ORIENTED_EDGE('',*,*,#4278,.F.);
#5279=ORIENTED_EDGE('',*,*,#4283,.F.);
#5280=ORIENTED_EDGE('',*,*,#4284,.T.);
#5281=ORIENTED_EDGE('',*,*,#4285,.F.);
#5282=ORIENTED_EDGE('',*,*,#4281,.F.);
#5283=ORIENTED_EDGE('',*,*,#4286,.F.);
#5284=ORIENTED_EDGE('',*,*,#4287,.T.);
#5285=ORIENTED_EDGE('',*,*,#4288,.F.);
#5286=ORIENTED_EDGE('',*,*,#4284,.F.);
#5287=ORIENTED_EDGE('',*,*,#4289,.F.);
#5288=ORIENTED_EDGE('',*,*,#4290,.T.);
#5289=ORIENTED_EDGE('',*,*,#4291,.F.);
#5290=ORIENTED_EDGE('',*,*,#4287,.F.);
#5291=ORIENTED_EDGE('',*,*,#4292,.F.);
#5292=ORIENTED_EDGE('',*,*,#4293,.T.);
#5293=ORIENTED_EDGE('',*,*,#4294,.F.);
#5294=ORIENTED_EDGE('',*,*,#4290,.F.);
#5295=ORIENTED_EDGE('',*,*,#4295,.F.);
#5296=ORIENTED_EDGE('',*,*,#4296,.T.);
#5297=ORIENTED_EDGE('',*,*,#4297,.F.);
#5298=ORIENTED_EDGE('',*,*,#4293,.F.);
#5299=ORIENTED_EDGE('',*,*,#4298,.F.);
#5300=ORIENTED_EDGE('',*,*,#4299,.F.);
#5301=ORIENTED_EDGE('',*,*,#4300,.F.);
#5302=ORIENTED_EDGE('',*,*,#4296,.F.);
#5303=ORIENTED_EDGE('',*,*,#4301,.F.);
#5304=ORIENTED_EDGE('',*,*,#4302,.T.);
#5305=ORIENTED_EDGE('',*,*,#4303,.F.);
#5306=ORIENTED_EDGE('',*,*,#4304,.F.);
#5307=ORIENTED_EDGE('',*,*,#4305,.F.);
#5308=ORIENTED_EDGE('',*,*,#4306,.T.);
#5309=ORIENTED_EDGE('',*,*,#4307,.F.);
#5310=ORIENTED_EDGE('',*,*,#4302,.F.);
#5311=ORIENTED_EDGE('',*,*,#4308,.F.);
#5312=ORIENTED_EDGE('',*,*,#4309,.T.);
#5313=ORIENTED_EDGE('',*,*,#4310,.F.);
#5314=ORIENTED_EDGE('',*,*,#4306,.F.);
#5315=ORIENTED_EDGE('',*,*,#4311,.F.);
#5316=ORIENTED_EDGE('',*,*,#4312,.T.);
#5317=ORIENTED_EDGE('',*,*,#4313,.F.);
#5318=ORIENTED_EDGE('',*,*,#4309,.F.);
#5319=ORIENTED_EDGE('',*,*,#4314,.F.);
#5320=ORIENTED_EDGE('',*,*,#4315,.T.);
#5321=ORIENTED_EDGE('',*,*,#4316,.F.);
#5322=ORIENTED_EDGE('',*,*,#4312,.F.);
#5323=ORIENTED_EDGE('',*,*,#4262,.T.);
#5324=ORIENTED_EDGE('',*,*,#4317,.F.);
#5325=ORIENTED_EDGE('',*,*,#4318,.T.);
#5326=ORIENTED_EDGE('',*,*,#4319,.F.);
#5327=ORIENTED_EDGE('',*,*,#4315,.F.);
#5328=ORIENTED_EDGE('',*,*,#4320,.F.);
#5329=ORIENTED_EDGE('',*,*,#4321,.T.);
#5330=ORIENTED_EDGE('',*,*,#4322,.F.);
#5331=ORIENTED_EDGE('',*,*,#4318,.F.);
#5332=ORIENTED_EDGE('',*,*,#4323,.F.);
#5333=ORIENTED_EDGE('',*,*,#4324,.T.);
#5334=ORIENTED_EDGE('',*,*,#4325,.F.);
#5335=ORIENTED_EDGE('',*,*,#4321,.F.);
#5336=ORIENTED_EDGE('',*,*,#4326,.F.);
#5337=ORIENTED_EDGE('',*,*,#4327,.F.);
#5338=ORIENTED_EDGE('',*,*,#4328,.F.);
#5339=ORIENTED_EDGE('',*,*,#4324,.F.);
#5340=ORIENTED_EDGE('',*,*,#4329,.F.);
#5341=ORIENTED_EDGE('',*,*,#4330,.T.);
#5342=ORIENTED_EDGE('',*,*,#4331,.F.);
#5343=ORIENTED_EDGE('',*,*,#4332,.F.);
#5344=ORIENTED_EDGE('',*,*,#4333,.F.);
#5345=ORIENTED_EDGE('',*,*,#4334,.T.);
#5346=ORIENTED_EDGE('',*,*,#4335,.F.);
#5347=ORIENTED_EDGE('',*,*,#4330,.F.);
#5348=ORIENTED_EDGE('',*,*,#4336,.F.);
#5349=ORIENTED_EDGE('',*,*,#4337,.T.);
#5350=ORIENTED_EDGE('',*,*,#4338,.F.);
#5351=ORIENTED_EDGE('',*,*,#4334,.F.);
#5352=ORIENTED_EDGE('',*,*,#4339,.F.);
#5353=ORIENTED_EDGE('',*,*,#4340,.T.);
#5354=ORIENTED_EDGE('',*,*,#4341,.F.);
#5355=ORIENTED_EDGE('',*,*,#4337,.F.);
#5356=ORIENTED_EDGE('',*,*,#4342,.F.);
#5357=ORIENTED_EDGE('',*,*,#4343,.T.);
#5358=ORIENTED_EDGE('',*,*,#4344,.F.);
#5359=ORIENTED_EDGE('',*,*,#4340,.F.);
#5360=ORIENTED_EDGE('',*,*,#4345,.F.);
#5361=ORIENTED_EDGE('',*,*,#4346,.T.);
#5362=ORIENTED_EDGE('',*,*,#4347,.F.);
#5363=ORIENTED_EDGE('',*,*,#4343,.F.);
#5364=ORIENTED_EDGE('',*,*,#4348,.F.);
#5365=ORIENTED_EDGE('',*,*,#4349,.T.);
#5366=ORIENTED_EDGE('',*,*,#4350,.F.);
#5367=ORIENTED_EDGE('',*,*,#4346,.F.);
#5368=ORIENTED_EDGE('',*,*,#4351,.F.);
#5369=ORIENTED_EDGE('',*,*,#4352,.T.);
#5370=ORIENTED_EDGE('',*,*,#4353,.F.);
#5371=ORIENTED_EDGE('',*,*,#4349,.F.);
#5372=ORIENTED_EDGE('',*,*,#4354,.F.);
#5373=ORIENTED_EDGE('',*,*,#4355,.F.);
#5374=ORIENTED_EDGE('',*,*,#4356,.F.);
#5375=ORIENTED_EDGE('',*,*,#4352,.F.);
#5376=ORIENTED_EDGE('',*,*,#4357,.F.);
#5377=ORIENTED_EDGE('',*,*,#4358,.T.);
#5378=ORIENTED_EDGE('',*,*,#4359,.F.);
#5379=ORIENTED_EDGE('',*,*,#4360,.F.);
#5380=ORIENTED_EDGE('',*,*,#4361,.F.);
#5381=ORIENTED_EDGE('',*,*,#4362,.T.);
#5382=ORIENTED_EDGE('',*,*,#4363,.F.);
#5383=ORIENTED_EDGE('',*,*,#4358,.F.);
#5384=ORIENTED_EDGE('',*,*,#4364,.F.);
#5385=ORIENTED_EDGE('',*,*,#4365,.T.);
#5386=ORIENTED_EDGE('',*,*,#4366,.F.);
#5387=ORIENTED_EDGE('',*,*,#4362,.F.);
#5388=ORIENTED_EDGE('',*,*,#4367,.F.);
#5389=ORIENTED_EDGE('',*,*,#4368,.T.);
#5390=ORIENTED_EDGE('',*,*,#4369,.F.);
#5391=ORIENTED_EDGE('',*,*,#4365,.F.);
#5392=ORIENTED_EDGE('',*,*,#4370,.F.);
#5393=ORIENTED_EDGE('',*,*,#4371,.T.);
#5394=ORIENTED_EDGE('',*,*,#4372,.F.);
#5395=ORIENTED_EDGE('',*,*,#4368,.F.);
#5396=ORIENTED_EDGE('',*,*,#4266,.T.);
#5397=ORIENTED_EDGE('',*,*,#4373,.F.);
#5398=ORIENTED_EDGE('',*,*,#4374,.T.);
#5399=ORIENTED_EDGE('',*,*,#4375,.F.);
#5400=ORIENTED_EDGE('',*,*,#4371,.F.);
#5401=ORIENTED_EDGE('',*,*,#4376,.F.);
#5402=ORIENTED_EDGE('',*,*,#4377,.T.);
#5403=ORIENTED_EDGE('',*,*,#4378,.F.);
#5404=ORIENTED_EDGE('',*,*,#4374,.F.);
#5405=ORIENTED_EDGE('',*,*,#4379,.F.);
#5406=ORIENTED_EDGE('',*,*,#4380,.T.);
#5407=ORIENTED_EDGE('',*,*,#4381,.F.);
#5408=ORIENTED_EDGE('',*,*,#4377,.F.);
#5409=ORIENTED_EDGE('',*,*,#4382,.F.);
#5410=ORIENTED_EDGE('',*,*,#4383,.F.);
#5411=ORIENTED_EDGE('',*,*,#4384,.F.);
#5412=ORIENTED_EDGE('',*,*,#4380,.F.);
#5413=ORIENTED_EDGE('',*,*,#4269,.T.);
#5414=ORIENTED_EDGE('',*,*,#4385,.T.);
#5415=ORIENTED_EDGE('',*,*,#4386,.F.);
#5416=ORIENTED_EDGE('',*,*,#4385,.F.);
#5417=ORIENTED_EDGE('',*,*,#4270,.T.);
#5418=ORIENTED_EDGE('',*,*,#4299,.T.);
#5419=ORIENTED_EDGE('',*,*,#4387,.T.);
#5420=ORIENTED_EDGE('',*,*,#4388,.T.);
#5421=ORIENTED_EDGE('',*,*,#4389,.F.);
#5422=ORIENTED_EDGE('',*,*,#4276,.T.);
#5423=ORIENTED_EDGE('',*,*,#4390,.F.);
#5424=ORIENTED_EDGE('',*,*,#4391,.F.);
#5425=ORIENTED_EDGE('',*,*,#4392,.T.);
#5426=ORIENTED_EDGE('',*,*,#4327,.T.);
#5427=ORIENTED_EDGE('',*,*,#4393,.T.);
#5428=ORIENTED_EDGE('',*,*,#4391,.T.);
#5429=ORIENTED_EDGE('',*,*,#4394,.F.);
#5430=ORIENTED_EDGE('',*,*,#4304,.T.);
#5431=ORIENTED_EDGE('',*,*,#4395,.F.);
#5432=ORIENTED_EDGE('',*,*,#4396,.F.);
#5433=ORIENTED_EDGE('',*,*,#4397,.T.);
#5434=ORIENTED_EDGE('',*,*,#4355,.T.);
#5435=ORIENTED_EDGE('',*,*,#4398,.T.);
#5436=ORIENTED_EDGE('',*,*,#4396,.T.);
#5437=ORIENTED_EDGE('',*,*,#4399,.F.);
#5438=ORIENTED_EDGE('',*,*,#4332,.T.);
#5439=ORIENTED_EDGE('',*,*,#4400,.F.);
#5440=ORIENTED_EDGE('',*,*,#4401,.F.);
#5441=ORIENTED_EDGE('',*,*,#4402,.T.);
#5442=ORIENTED_EDGE('',*,*,#4383,.T.);
#5443=ORIENTED_EDGE('',*,*,#4403,.T.);
#5444=ORIENTED_EDGE('',*,*,#4401,.T.);
#5445=ORIENTED_EDGE('',*,*,#4404,.F.);
#5446=ORIENTED_EDGE('',*,*,#4360,.T.);
#5447=ORIENTED_EDGE('',*,*,#4405,.F.);
#5448=ORIENTED_EDGE('',*,*,#4388,.F.);
#5449=ORIENTED_EDGE('',*,*,#4406,.T.);
#5450=ORIENTED_EDGE('',*,*,#4275,.T.);
#5451=ORIENTED_EDGE('',*,*,#4279,.T.);
#5452=ORIENTED_EDGE('',*,*,#4282,.T.);
#5453=ORIENTED_EDGE('',*,*,#4285,.T.);
#5454=ORIENTED_EDGE('',*,*,#4288,.T.);
#5455=ORIENTED_EDGE('',*,*,#4291,.T.);
#5456=ORIENTED_EDGE('',*,*,#4294,.T.);
#5457=ORIENTED_EDGE('',*,*,#4297,.T.);
#5458=ORIENTED_EDGE('',*,*,#4300,.T.);
#5459=ORIENTED_EDGE('',*,*,#4389,.T.);
#5460=ORIENTED_EDGE('',*,*,#4405,.T.);
#5461=ORIENTED_EDGE('',*,*,#4359,.T.);
#5462=ORIENTED_EDGE('',*,*,#4363,.T.);
#5463=ORIENTED_EDGE('',*,*,#4366,.T.);
#5464=ORIENTED_EDGE('',*,*,#4369,.T.);
#5465=ORIENTED_EDGE('',*,*,#4372,.T.);
#5466=ORIENTED_EDGE('',*,*,#4375,.T.);
#5467=ORIENTED_EDGE('',*,*,#4378,.T.);
#5468=ORIENTED_EDGE('',*,*,#4381,.T.);
#5469=ORIENTED_EDGE('',*,*,#4384,.T.);
#5470=ORIENTED_EDGE('',*,*,#4404,.T.);
#5471=ORIENTED_EDGE('',*,*,#4400,.T.);
#5472=ORIENTED_EDGE('',*,*,#4331,.T.);
#5473=ORIENTED_EDGE('',*,*,#4335,.T.);
#5474=ORIENTED_EDGE('',*,*,#4338,.T.);
#5475=ORIENTED_EDGE('',*,*,#4341,.T.);
#5476=ORIENTED_EDGE('',*,*,#4344,.T.);
#5477=ORIENTED_EDGE('',*,*,#4347,.T.);
#5478=ORIENTED_EDGE('',*,*,#4350,.T.);
#5479=ORIENTED_EDGE('',*,*,#4353,.T.);
#5480=ORIENTED_EDGE('',*,*,#4356,.T.);
#5481=ORIENTED_EDGE('',*,*,#4399,.T.);
#5482=ORIENTED_EDGE('',*,*,#4395,.T.);
#5483=ORIENTED_EDGE('',*,*,#4303,.T.);
#5484=ORIENTED_EDGE('',*,*,#4307,.T.);
#5485=ORIENTED_EDGE('',*,*,#4310,.T.);
#5486=ORIENTED_EDGE('',*,*,#4313,.T.);
#5487=ORIENTED_EDGE('',*,*,#4316,.T.);
#5488=ORIENTED_EDGE('',*,*,#4319,.T.);
#5489=ORIENTED_EDGE('',*,*,#4322,.T.);
#5490=ORIENTED_EDGE('',*,*,#4325,.T.);
#5491=ORIENTED_EDGE('',*,*,#4328,.T.);
#5492=ORIENTED_EDGE('',*,*,#4394,.T.);
#5493=ORIENTED_EDGE('',*,*,#4390,.T.);
#5494=ORIENTED_EDGE('',*,*,#4386,.T.);
#5495=ORIENTED_EDGE('',*,*,#4273,.T.);
#5496=ORIENTED_EDGE('',*,*,#4392,.F.);
#5497=ORIENTED_EDGE('',*,*,#4393,.F.);
#5498=ORIENTED_EDGE('',*,*,#4326,.T.);
#5499=ORIENTED_EDGE('',*,*,#4323,.T.);
#5500=ORIENTED_EDGE('',*,*,#4320,.T.);
#5501=ORIENTED_EDGE('',*,*,#4317,.T.);
#5502=ORIENTED_EDGE('',*,*,#4314,.T.);
#5503=ORIENTED_EDGE('',*,*,#4311,.T.);
#5504=ORIENTED_EDGE('',*,*,#4308,.T.);
#5505=ORIENTED_EDGE('',*,*,#4305,.T.);
#5506=ORIENTED_EDGE('',*,*,#4301,.T.);
#5507=ORIENTED_EDGE('',*,*,#4397,.F.);
#5508=ORIENTED_EDGE('',*,*,#4398,.F.);
#5509=ORIENTED_EDGE('',*,*,#4354,.T.);
#5510=ORIENTED_EDGE('',*,*,#4351,.T.);
#5511=ORIENTED_EDGE('',*,*,#4348,.T.);
#5512=ORIENTED_EDGE('',*,*,#4345,.T.);
#5513=ORIENTED_EDGE('',*,*,#4342,.T.);
#5514=ORIENTED_EDGE('',*,*,#4339,.T.);
#5515=ORIENTED_EDGE('',*,*,#4336,.T.);
#5516=ORIENTED_EDGE('',*,*,#4333,.T.);
#5517=ORIENTED_EDGE('',*,*,#4329,.T.);
#5518=ORIENTED_EDGE('',*,*,#4402,.F.);
#5519=ORIENTED_EDGE('',*,*,#4403,.F.);
#5520=ORIENTED_EDGE('',*,*,#4382,.T.);
#5521=ORIENTED_EDGE('',*,*,#4379,.T.);
#5522=ORIENTED_EDGE('',*,*,#4376,.T.);
#5523=ORIENTED_EDGE('',*,*,#4373,.T.);
#5524=ORIENTED_EDGE('',*,*,#4370,.T.);
#5525=ORIENTED_EDGE('',*,*,#4367,.T.);
#5526=ORIENTED_EDGE('',*,*,#4364,.T.);
#5527=ORIENTED_EDGE('',*,*,#4361,.T.);
#5528=ORIENTED_EDGE('',*,*,#4357,.T.);
#5529=ORIENTED_EDGE('',*,*,#4406,.F.);
#5530=ORIENTED_EDGE('',*,*,#4387,.F.);
#5531=ORIENTED_EDGE('',*,*,#4298,.T.);
#5532=ORIENTED_EDGE('',*,*,#4295,.T.);
#5533=ORIENTED_EDGE('',*,*,#4292,.T.);
#5534=ORIENTED_EDGE('',*,*,#4289,.T.);
#5535=ORIENTED_EDGE('',*,*,#4286,.T.);
#5536=ORIENTED_EDGE('',*,*,#4283,.T.);
#5537=ORIENTED_EDGE('',*,*,#4280,.T.);
#5538=ORIENTED_EDGE('',*,*,#4277,.T.);
#5539=ORIENTED_EDGE('',*,*,#4271,.T.);
#7134=CYLINDRICAL_SURFACE('',#8070,0.275);
#7135=CYLINDRICAL_SURFACE('',#8073,0.21);
#7136=CYLINDRICAL_SURFACE('',#8111,0.21);
#7218=ADVANCED_FACE('',(#1017,#617),#7134,.F.);
#7219=ADVANCED_FACE('',(#1018),#7135,.F.);
#7220=ADVANCED_FACE('',(#1019),#708,.F.);
#7221=ADVANCED_FACE('',(#1020),#709,.F.);
#7222=ADVANCED_FACE('',(#1021),#710,.F.);
#7223=ADVANCED_FACE('',(#1022),#711,.F.);
#7224=ADVANCED_FACE('',(#1023),#712,.F.);
#7225=ADVANCED_FACE('',(#1024),#713,.F.);
#7226=ADVANCED_FACE('',(#1025),#714,.F.);
#7227=ADVANCED_FACE('',(#1026),#715,.F.);
#7228=ADVANCED_FACE('',(#1027),#716,.F.);
#7229=ADVANCED_FACE('',(#1028),#717,.F.);
#7230=ADVANCED_FACE('',(#1029),#718,.F.);
#7231=ADVANCED_FACE('',(#1030),#719,.F.);
#7232=ADVANCED_FACE('',(#1031),#720,.F.);
#7233=ADVANCED_FACE('',(#1032,#618),#721,.F.);
#7234=ADVANCED_FACE('',(#1033),#722,.F.);
#7235=ADVANCED_FACE('',(#1034),#723,.F.);
#7236=ADVANCED_FACE('',(#1035),#724,.F.);
#7237=ADVANCED_FACE('',(#1036),#725,.F.);
#7238=ADVANCED_FACE('',(#1037),#726,.F.);
#7239=ADVANCED_FACE('',(#1038),#727,.F.);
#7240=ADVANCED_FACE('',(#1039),#728,.F.);
#7241=ADVANCED_FACE('',(#1040),#729,.F.);
#7242=ADVANCED_FACE('',(#1041),#730,.F.);
#7243=ADVANCED_FACE('',(#1042),#731,.F.);
#7244=ADVANCED_FACE('',(#1043),#732,.F.);
#7245=ADVANCED_FACE('',(#1044),#733,.F.);
#7246=ADVANCED_FACE('',(#1045),#734,.F.);
#7247=ADVANCED_FACE('',(#1046),#735,.F.);
#7248=ADVANCED_FACE('',(#1047),#736,.F.);
#7249=ADVANCED_FACE('',(#1048),#737,.F.);
#7250=ADVANCED_FACE('',(#1049),#738,.F.);
#7251=ADVANCED_FACE('',(#1050,#619),#739,.F.);
#7252=ADVANCED_FACE('',(#1051),#740,.F.);
#7253=ADVANCED_FACE('',(#1052),#741,.F.);
#7254=ADVANCED_FACE('',(#1053),#742,.F.);
#7255=ADVANCED_FACE('',(#1054),#743,.F.);
#7256=ADVANCED_FACE('',(#1055),#7136,.F.);
#7257=ADVANCED_FACE('',(#1056),#744,.T.);
#7258=ADVANCED_FACE('',(#1057),#745,.T.);
#7259=ADVANCED_FACE('',(#1058),#746,.T.);
#7260=ADVANCED_FACE('',(#1059),#747,.T.);
#7261=ADVANCED_FACE('',(#1060),#748,.T.);
#7262=ADVANCED_FACE('',(#1061),#749,.T.);
#7263=ADVANCED_FACE('',(#1062),#750,.T.);
#7264=ADVANCED_FACE('',(#1063),#751,.T.);
#7265=ADVANCED_FACE('',(#1064,#620),#752,.T.);
#7266=ADVANCED_FACE('',(#1065,#621),#753,.F.);
#7628=CLOSED_SHELL('',(#7218,#7219,#7220,#7221,#7222,#7223,#7224,#7225,
#7226,#7227,#7228,#7229,#7230,#7231,#7232,#7233,#7234,#7235,#7236,#7237,
#7238,#7239,#7240,#7241,#7242,#7243,#7244,#7245,#7246,#7247,#7248,#7249,
#7250,#7251,#7252,#7253,#7254,#7255,#7256,#7257,#7258,#7259,#7260,#7261,
#7262,#7263,#7264,#7265,#7266));
#8069=AXIS2_PLACEMENT_3D('',#11126,#8875,#8876);
#8070=AXIS2_PLACEMENT_3D('',#11127,#8877,#8878);
#8071=AXIS2_PLACEMENT_3D('',#11129,#8879,#8880);
#8072=AXIS2_PLACEMENT_3D('',#11157,#8883,#8884);
#8073=AXIS2_PLACEMENT_3D('',#11229,#8885,#8886);
#8074=AXIS2_PLACEMENT_3D('',#11231,#8887,#8888);
#8075=AXIS2_PLACEMENT_3D('',#11233,#8890,#8891);
#8076=AXIS2_PLACEMENT_3D('',#11242,#8896,#8897);
#8077=AXIS2_PLACEMENT_3D('',#11248,#8901,#8902);
#8078=AXIS2_PLACEMENT_3D('',#11254,#8906,#8907);
#8079=AXIS2_PLACEMENT_3D('',#11260,#8911,#8912);
#8080=AXIS2_PLACEMENT_3D('',#11266,#8916,#8917);
#8081=AXIS2_PLACEMENT_3D('',#11272,#8921,#8922);
#8082=AXIS2_PLACEMENT_3D('',#11278,#8926,#8927);
#8083=AXIS2_PLACEMENT_3D('',#11284,#8931,#8932);
#8084=AXIS2_PLACEMENT_3D('',#11290,#8936,#8937);
#8085=AXIS2_PLACEMENT_3D('',#11299,#8942,#8943);
#8086=AXIS2_PLACEMENT_3D('',#11305,#8947,#8948);
#8087=AXIS2_PLACEMENT_3D('',#11311,#8952,#8953);
#8088=AXIS2_PLACEMENT_3D('',#11317,#8957,#8958);
#8089=AXIS2_PLACEMENT_3D('',#11323,#8962,#8963);
#8090=AXIS2_PLACEMENT_3D('',#11329,#8967,#8968);
#8091=AXIS2_PLACEMENT_3D('',#11335,#8972,#8973);
#8092=AXIS2_PLACEMENT_3D('',#11341,#8977,#8978);
#8093=AXIS2_PLACEMENT_3D('',#11347,#8982,#8983);
#8094=AXIS2_PLACEMENT_3D('',#11356,#8988,#8989);
#8095=AXIS2_PLACEMENT_3D('',#11362,#8993,#8994);
#8096=AXIS2_PLACEMENT_3D('',#11368,#8998,#8999);
#8097=AXIS2_PLACEMENT_3D('',#11374,#9003,#9004);
#8098=AXIS2_PLACEMENT_3D('',#11380,#9008,#9009);
#8099=AXIS2_PLACEMENT_3D('',#11386,#9013,#9014);
#8100=AXIS2_PLACEMENT_3D('',#11392,#9018,#9019);
#8101=AXIS2_PLACEMENT_3D('',#11398,#9023,#9024);
#8102=AXIS2_PLACEMENT_3D('',#11404,#9028,#9029);
#8103=AXIS2_PLACEMENT_3D('',#11413,#9034,#9035);
#8104=AXIS2_PLACEMENT_3D('',#11419,#9039,#9040);
#8105=AXIS2_PLACEMENT_3D('',#11425,#9044,#9045);
#8106=AXIS2_PLACEMENT_3D('',#11431,#9049,#9050);
#8107=AXIS2_PLACEMENT_3D('',#11437,#9054,#9055);
#8108=AXIS2_PLACEMENT_3D('',#11443,#9059,#9060);
#8109=AXIS2_PLACEMENT_3D('',#11449,#9064,#9065);
#8110=AXIS2_PLACEMENT_3D('',#11455,#9069,#9070);
#8111=AXIS2_PLACEMENT_3D('',#11461,#9074,#9075);
#8112=AXIS2_PLACEMENT_3D('',#11464,#9077,#9078);
#8113=AXIS2_PLACEMENT_3D('',#11465,#9079,#9080);
#8114=AXIS2_PLACEMENT_3D('',#11471,#9084,#9085);
#8115=AXIS2_PLACEMENT_3D('',#11477,#9089,#9090);
#8116=AXIS2_PLACEMENT_3D('',#11480,#9093,#9094);
#8117=AXIS2_PLACEMENT_3D('',#11486,#9098,#9099);
#8118=AXIS2_PLACEMENT_3D('',#11489,#9102,#9103);
#8119=AXIS2_PLACEMENT_3D('',#11495,#9107,#9108);
#8120=AXIS2_PLACEMENT_3D('',#11498,#9111,#9112);
#8121=AXIS2_PLACEMENT_3D('',#11501,#9115,#9116);
#8122=AXIS2_PLACEMENT_3D('',#11502,#9117,#9118);
#8875=DIRECTION('axis',(0.,0.,1.));
#8876=DIRECTION('refdir',(1.,0.,0.));
#8877=DIRECTION('center_axis',(0.,0.,1.));
#8878=DIRECTION('ref_axis',(1.,0.,0.));
#8879=DIRECTION('center_axis',(0.,0.,1.));
#8880=DIRECTION('ref_axis',(1.,0.,0.));
#8881=DIRECTION('',(0.,0.,1.));
#8882=DIRECTION('',(0.,0.,1.));
#8883=DIRECTION('center_axis',(0.,0.,-1.));
#8884=DIRECTION('ref_axis',(1.,0.,0.));
#8885=DIRECTION('center_axis',(1.,0.,0.));
#8886=DIRECTION('ref_axis',(0.,0.,-1.));
#8887=DIRECTION('center_axis',(1.,0.,0.));
#8888=DIRECTION('ref_axis',(0.,0.,-1.));
#8889=DIRECTION('',(1.,0.,0.));
#8890=DIRECTION('center_axis',(0.,0.,-1.));
#8891=DIRECTION('ref_axis',(0.,1.,0.));
#8892=DIRECTION('',(0.,1.,0.));
#8893=DIRECTION('',(1.,0.,0.));
#8894=DIRECTION('',(0.,-1.,0.));
#8895=DIRECTION('',(1.,0.,0.));
#8896=DIRECTION('center_axis',(0.,1.,-8.88178419700125E-16));
#8897=DIRECTION('ref_axis',(0.,8.88178419700125E-16,1.));
#8898=DIRECTION('',(0.,8.88178419700125E-16,1.));
#8899=DIRECTION('',(1.,0.,0.));
#8900=DIRECTION('',(0.,-8.88178419700125E-16,-1.));
#8901=DIRECTION('center_axis',(0.,-7.40148683083439E-16,-1.));
#8902=DIRECTION('ref_axis',(0.,1.,-7.40148683083439E-16));
#8903=DIRECTION('',(0.,1.,-7.40148683083439E-16));
#8904=DIRECTION('',(1.,0.,0.));
#8905=DIRECTION('',(0.,-1.,7.40148683083439E-16));
#8906=DIRECTION('center_axis',(0.,-0.707106781186547,-0.707106781186548));
#8907=DIRECTION('ref_axis',(0.,0.707106781186548,-0.707106781186547));
#8908=DIRECTION('',(0.,0.707106781186548,-0.707106781186547));
#8909=DIRECTION('',(1.,0.,0.));
#8910=DIRECTION('',(0.,-0.707106781186548,0.707106781186547));
#8911=DIRECTION('center_axis',(0.,-1.,2.77555756156289E-16));
#8912=DIRECTION('ref_axis',(0.,-2.77555756156289E-16,-1.));
#8913=DIRECTION('',(0.,-2.77555756156289E-16,-1.));
#8914=DIRECTION('',(1.,0.,0.));
#8915=DIRECTION('',(0.,2.77555756156289E-16,1.));
#8916=DIRECTION('center_axis',(0.,-0.707106781186547,0.707106781186548));
#8917=DIRECTION('ref_axis',(0.,-0.707106781186548,-0.707106781186547));
#8918=DIRECTION('',(0.,-0.707106781186548,-0.707106781186547));
#8919=DIRECTION('',(1.,0.,0.));
#8920=DIRECTION('',(0.,0.707106781186548,0.707106781186547));
#8921=DIRECTION('center_axis',(0.,7.40148683083438E-16,1.));
#8922=DIRECTION('ref_axis',(0.,-1.,7.40148683083438E-16));
#8923=DIRECTION('',(0.,-1.,7.40148683083438E-16));
#8924=DIRECTION('',(1.,0.,0.));
#8925=DIRECTION('',(0.,1.,-7.40148683083438E-16));
#8926=DIRECTION('center_axis',(0.,1.,-4.44089209850063E-16));
#8927=DIRECTION('ref_axis',(0.,4.44089209850063E-16,1.));
#8928=DIRECTION('',(0.,4.44089209850063E-16,1.));
#8929=DIRECTION('',(1.,0.,0.));
#8930=DIRECTION('',(0.,-4.44089209850063E-16,-1.));
#8931=DIRECTION('center_axis',(0.,2.41352831440251E-16,1.));
#8932=DIRECTION('ref_axis',(0.,-1.,2.41352831440251E-16));
#8933=DIRECTION('',(0.,-1.,2.41352831440251E-16));
#8934=DIRECTION('',(-1.,0.,0.));
#8935=DIRECTION('',(0.,1.,-2.41352831440251E-16));
#8936=DIRECTION('center_axis',(0.,-1.,2.41352831440251E-16));
#8937=DIRECTION('ref_axis',(0.,-2.41352831440251E-16,-1.));
#8938=DIRECTION('',(0.,-2.41352831440251E-16,-1.));
#8939=DIRECTION('',(1.,0.,0.));
#8940=DIRECTION('',(0.,2.41352831440251E-16,1.));
#8941=DIRECTION('',(1.,0.,0.));
#8942=DIRECTION('center_axis',(0.,0.,-1.));
#8943=DIRECTION('ref_axis',(0.,1.,0.));
#8944=DIRECTION('',(0.,1.,0.));
#8945=DIRECTION('',(1.,0.,0.));
#8946=DIRECTION('',(0.,-1.,0.));
#8947=DIRECTION('center_axis',(0.,-1.,0.));
#8948=DIRECTION('ref_axis',(0.,0.,-1.));
#8949=DIRECTION('',(0.,0.,-1.));
#8950=DIRECTION('',(1.,0.,0.));
#8951=DIRECTION('',(0.,0.,1.));
#8952=DIRECTION('center_axis',(0.,-0.707106781186547,0.707106781186548));
#8953=DIRECTION('ref_axis',(0.,-0.707106781186548,-0.707106781186547));
#8954=DIRECTION('',(0.,-0.707106781186548,-0.707106781186547));
#8955=DIRECTION('',(1.,0.,0.));
#8956=DIRECTION('',(0.,0.707106781186548,0.707106781186547));
#8957=DIRECTION('center_axis',(0.,0.,1.));
#8958=DIRECTION('ref_axis',(0.,-1.,0.));
#8959=DIRECTION('',(0.,-1.,0.));
#8960=DIRECTION('',(1.,0.,0.));
#8961=DIRECTION('',(0.,1.,0.));
#8962=DIRECTION('center_axis',(0.,0.707106781186548,0.707106781186547));
#8963=DIRECTION('ref_axis',(0.,-0.707106781186547,0.707106781186548));
#8964=DIRECTION('',(0.,-0.707106781186547,0.707106781186548));
#8965=DIRECTION('',(1.,0.,0.));
#8966=DIRECTION('',(0.,0.707106781186547,-0.707106781186548));
#8967=DIRECTION('center_axis',(0.,1.,0.));
#8968=DIRECTION('ref_axis',(0.,0.,1.));
#8969=DIRECTION('',(0.,0.,1.));
#8970=DIRECTION('',(1.,0.,0.));
#8971=DIRECTION('',(0.,0.,-1.));
#8972=DIRECTION('center_axis',(0.,0.,-1.));
#8973=DIRECTION('ref_axis',(0.,1.,0.));
#8974=DIRECTION('',(0.,1.,0.));
#8975=DIRECTION('',(1.,0.,0.));
#8976=DIRECTION('',(0.,-1.,0.));
#8977=DIRECTION('center_axis',(0.,1.,-2.41352831440251E-16));
#8978=DIRECTION('ref_axis',(0.,2.41352831440251E-16,1.));
#8979=DIRECTION('',(0.,2.41352831440251E-16,1.));
#8980=DIRECTION('',(-1.,0.,0.));
#8981=DIRECTION('',(0.,-2.41352831440251E-16,-1.));
#8982=DIRECTION('center_axis',(0.,0.,1.));
#8983=DIRECTION('ref_axis',(0.,-1.,0.));
#8984=DIRECTION('',(0.,-1.,0.));
#8985=DIRECTION('',(1.,0.,0.));
#8986=DIRECTION('',(0.,1.,0.));
#8987=DIRECTION('',(1.,0.,0.));
#8988=DIRECTION('center_axis',(0.,-1.,0.));
#8989=DIRECTION('ref_axis',(0.,0.,-1.));
#8990=DIRECTION('',(0.,0.,-1.));
#8991=DIRECTION('',(1.,0.,0.));
#8992=DIRECTION('',(0.,0.,1.));
#8993=DIRECTION('center_axis',(0.,0.,1.));
#8994=DIRECTION('ref_axis',(0.,-1.,0.));
#8995=DIRECTION('',(0.,-1.,0.));
#8996=DIRECTION('',(1.,0.,0.));
#8997=DIRECTION('',(0.,1.,0.));
#8998=DIRECTION('center_axis',(0.,0.707106781186548,0.707106781186548));
#8999=DIRECTION('ref_axis',(0.,-0.707106781186548,0.707106781186548));
#9000=DIRECTION('',(0.,-0.707106781186548,0.707106781186548));
#9001=DIRECTION('',(1.,0.,0.));
#9002=DIRECTION('',(0.,0.707106781186548,-0.707106781186548));
#9003=DIRECTION('center_axis',(0.,1.,0.));
#9004=DIRECTION('ref_axis',(0.,0.,1.));
#9005=DIRECTION('',(0.,0.,1.));
#9006=DIRECTION('',(1.,0.,0.));
#9007=DIRECTION('',(0.,0.,-1.));
#9008=DIRECTION('center_axis',(0.,0.707106781186548,-0.707106781186547));
#9009=DIRECTION('ref_axis',(0.,0.707106781186547,0.707106781186548));
#9010=DIRECTION('',(0.,0.707106781186547,0.707106781186548));
#9011=DIRECTION('',(1.,0.,0.));
#9012=DIRECTION('',(0.,-0.707106781186547,-0.707106781186548));
#9013=DIRECTION('center_axis',(0.,-7.40148683083438E-16,-1.));
#9014=DIRECTION('ref_axis',(0.,1.,-7.40148683083438E-16));
#9015=DIRECTION('',(0.,1.,-7.40148683083438E-16));
#9016=DIRECTION('',(1.,0.,0.));
#9017=DIRECTION('',(0.,-1.,7.40148683083438E-16));
#9018=DIRECTION('center_axis',(0.,-1.,0.));
#9019=DIRECTION('ref_axis',(0.,0.,-1.));
#9020=DIRECTION('',(0.,0.,-1.));
#9021=DIRECTION('',(1.,0.,0.));
#9022=DIRECTION('',(0.,0.,1.));
#9023=DIRECTION('center_axis',(0.,0.,-1.));
#9024=DIRECTION('ref_axis',(0.,1.,0.));
#9025=DIRECTION('',(0.,1.,0.));
#9026=DIRECTION('',(-1.,0.,0.));
#9027=DIRECTION('',(0.,-1.,0.));
#9028=DIRECTION('center_axis',(0.,1.,0.));
#9029=DIRECTION('ref_axis',(0.,0.,1.));
#9030=DIRECTION('',(0.,0.,1.));
#9031=DIRECTION('',(1.,0.,0.));
#9032=DIRECTION('',(0.,0.,-1.));
#9033=DIRECTION('',(1.,0.,0.));
#9034=DIRECTION('center_axis',(0.,0.,1.));
#9035=DIRECTION('ref_axis',(0.,-1.,0.));
#9036=DIRECTION('',(0.,-1.,0.));
#9037=DIRECTION('',(1.,0.,0.));
#9038=DIRECTION('',(0.,1.,0.));
#9039=DIRECTION('center_axis',(0.,1.,0.));
#9040=DIRECTION('ref_axis',(0.,0.,1.));
#9041=DIRECTION('',(0.,0.,1.));
#9042=DIRECTION('',(1.,0.,0.));
#9043=DIRECTION('',(0.,0.,-1.));
#9044=DIRECTION('center_axis',(0.,0.707106781186547,-0.707106781186548));
#9045=DIRECTION('ref_axis',(0.,0.707106781186548,0.707106781186547));
#9046=DIRECTION('',(0.,0.707106781186548,0.707106781186547));
#9047=DIRECTION('',(1.,0.,0.));
#9048=DIRECTION('',(0.,-0.707106781186548,-0.707106781186547));
#9049=DIRECTION('center_axis',(0.,0.,-1.));
#9050=DIRECTION('ref_axis',(0.,1.,0.));
#9051=DIRECTION('',(0.,1.,0.));
#9052=DIRECTION('',(1.,0.,0.));
#9053=DIRECTION('',(0.,-1.,0.));
#9054=DIRECTION('center_axis',(0.,-0.707106781186547,-0.707106781186548));
#9055=DIRECTION('ref_axis',(0.,0.707106781186548,-0.707106781186547));
#9056=DIRECTION('',(0.,0.707106781186548,-0.707106781186547));
#9057=DIRECTION('',(1.,0.,0.));
#9058=DIRECTION('',(0.,-0.707106781186548,0.707106781186547));
#9059=DIRECTION('center_axis',(0.,-1.,0.));
#9060=DIRECTION('ref_axis',(0.,0.,-1.));
#9061=DIRECTION('',(0.,0.,-1.));
#9062=DIRECTION('',(1.,0.,0.));
#9063=DIRECTION('',(0.,0.,1.));
#9064=DIRECTION('center_axis',(0.,0.,1.));
#9065=DIRECTION('ref_axis',(0.,-1.,0.));
#9066=DIRECTION('',(0.,-1.,0.));
#9067=DIRECTION('',(1.,0.,0.));
#9068=DIRECTION('',(0.,1.,0.));
#9069=DIRECTION('center_axis',(0.,-1.,0.));
#9070=DIRECTION('ref_axis',(0.,0.,-1.));
#9071=DIRECTION('',(0.,0.,-1.));
#9072=DIRECTION('',(-1.,0.,0.));
#9073=DIRECTION('',(0.,0.,1.));
#9074=DIRECTION('center_axis',(1.,0.,0.));
#9075=DIRECTION('ref_axis',(0.,0.,-1.));
#9076=DIRECTION('',(1.,0.,0.));
#9077=DIRECTION('center_axis',(-1.,0.,0.));
#9078=DIRECTION('ref_axis',(0.,0.,-1.));
#9079=DIRECTION('center_axis',(0.,1.,0.));
#9080=DIRECTION('ref_axis',(0.,0.,1.));
#9081=DIRECTION('',(0.,0.,1.));
#9082=DIRECTION('',(1.,0.,0.));
#9083=DIRECTION('',(0.,0.,1.));
#9084=DIRECTION('center_axis',(0.,1.,0.));
#9085=DIRECTION('ref_axis',(0.,0.,1.));
#9086=DIRECTION('',(0.,0.,1.));
#9087=DIRECTION('',(1.,0.,0.));
#9088=DIRECTION('',(0.,0.,1.));
#9089=DIRECTION('center_axis',(0.,0.,-1.));
#9090=DIRECTION('ref_axis',(0.,1.,0.));
#9091=DIRECTION('',(0.,1.,0.));
#9092=DIRECTION('',(0.,1.,0.));
#9093=DIRECTION('center_axis',(0.,0.,-1.));
#9094=DIRECTION('ref_axis',(0.,1.,0.));
#9095=DIRECTION('',(0.,1.,0.));
#9096=DIRECTION('',(1.,0.,0.));
#9097=DIRECTION('',(0.,1.,0.));
#9098=DIRECTION('center_axis',(0.,-1.,0.));
#9099=DIRECTION('ref_axis',(0.,0.,-1.));
#9100=DIRECTION('',(0.,0.,-1.));
#9101=DIRECTION('',(0.,0.,-1.));
#9102=DIRECTION('center_axis',(0.,-1.,0.));
#9103=DIRECTION('ref_axis',(0.,0.,-1.));
#9104=DIRECTION('',(0.,0.,-1.));
#9105=DIRECTION('',(1.,0.,0.));
#9106=DIRECTION('',(0.,0.,-1.));
#9107=DIRECTION('center_axis',(0.,0.,1.));
#9108=DIRECTION('ref_axis',(0.,-1.,0.));
#9109=DIRECTION('',(0.,-1.,0.));
#9110=DIRECTION('',(0.,-1.,0.));
#9111=DIRECTION('center_axis',(0.,0.,1.));
#9112=DIRECTION('ref_axis',(0.,-1.,0.));
#9113=DIRECTION('',(0.,-1.,0.));
#9114=DIRECTION('',(0.,-1.,0.));
#9115=DIRECTION('center_axis',(1.,0.,0.));
#9116=DIRECTION('ref_axis',(0.,0.,-1.));
#9117=DIRECTION('center_axis',(1.,0.,0.));
#9118=DIRECTION('ref_axis',(0.,0.,-1.));
#11126=CARTESIAN_POINT('',(0.,0.,0.));
#11127=CARTESIAN_POINT('Origin',(6.,0.,-1.1));
#11128=CARTESIAN_POINT('',(5.725,-3.36777869765523E-17,-0.42));
#11129=CARTESIAN_POINT('Origin',(6.,0.,-0.42));
#11130=CARTESIAN_POINT('',(5.725,-4.4594469103905E-17,-0.21));
#11131=CARTESIAN_POINT('',(5.725,-3.36777869765523E-17,-1.1));
#11132=CARTESIAN_POINT('',(5.725,3.97778822344556E-18,0.21));
#11133=CARTESIAN_POINT('Ctrl Pts',(5.725,3.81639164714898E-17,0.21));
#11134=CARTESIAN_POINT('Ctrl Pts',(5.725,-0.027663639322611,0.21));
#11135=CARTESIAN_POINT('Ctrl Pts',(5.72949374752355,-0.0563806217319961,
0.204214038345313));
#11136=CARTESIAN_POINT('Ctrl Pts',(5.74560158587233,-0.107860332287473,
0.182341144032028));
#11137=CARTESIAN_POINT('Ctrl Pts',(5.75710894103549,-0.130678518444188,
0.166306329654162));
#11138=CARTESIAN_POINT('Ctrl Pts',(5.78023922617715,-0.166732877511574,
0.130251970586776));
#11139=CARTESIAN_POINT('Ctrl Pts',(5.7937414503193,-0.182517999394844,0.107475484252794));
#11140=CARTESIAN_POINT('Ctrl Pts',(5.80974723471181,-0.198712082533353,
0.0693141634661022));
#11141=CARTESIAN_POINT('Ctrl Pts',(5.81433611385285,-0.202908887997328,
0.0559106681449083));
#11142=CARTESIAN_POINT('Ctrl Pts',(5.82070090566933,-0.208554382393535,
0.0283388251429182));
#11143=CARTESIAN_POINT('Ctrl Pts',(5.82244719095435,-0.21,0.0141630178371274));
#11144=CARTESIAN_POINT('Ctrl Pts',(5.82244719095435,-0.21,-0.0141630178371274));
#11145=CARTESIAN_POINT('Ctrl Pts',(5.82070090566933,-0.208554382393535,
-0.0283388251429182));
#11146=CARTESIAN_POINT('Ctrl Pts',(5.81433611385285,-0.202908887997328,
-0.0559106681449083));
#11147=CARTESIAN_POINT('Ctrl Pts',(5.80974723471181,-0.198712082533353,
-0.0693141634661022));
#11148=CARTESIAN_POINT('Ctrl Pts',(5.7937414503193,-0.182517999394844,-0.107475484252795));
#11149=CARTESIAN_POINT('Ctrl Pts',(5.78023922617715,-0.166732877511574,
-0.130251970586776));
#11150=CARTESIAN_POINT('Ctrl Pts',(5.75710894103549,-0.130678518444188,
-0.166306329654162));
#11151=CARTESIAN_POINT('Ctrl Pts',(5.74560158587233,-0.107860332287473,
-0.182341144032028));
#11152=CARTESIAN_POINT('Ctrl Pts',(5.72949374752355,-0.0563806217319961,
-0.204214038345313));
#11153=CARTESIAN_POINT('Ctrl Pts',(5.725,-0.0276636393226111,-0.21));
#11154=CARTESIAN_POINT('Ctrl Pts',(5.725,-5.55111512312578E-17,-0.21));
#11155=CARTESIAN_POINT('',(5.725,3.36777869765523E-17,0.42));
#11156=CARTESIAN_POINT('',(5.725,-3.36777869765523E-17,-1.1));
#11157=CARTESIAN_POINT('Origin',(6.,0.,0.42));
#11158=CARTESIAN_POINT('',(5.82244719095435,0.21,2.25514051876985E-17));
#11159=CARTESIAN_POINT('Ctrl Pts',(5.82244719095435,0.21,2.25514051876985E-17));
#11160=CARTESIAN_POINT('Ctrl Pts',(5.82244719095435,0.21,0.0141630178371274));
#11161=CARTESIAN_POINT('Ctrl Pts',(5.82070090566933,0.208554382393535,0.0283388251429182));
#11162=CARTESIAN_POINT('Ctrl Pts',(5.81433611385285,0.202908887997328,0.0559106681449083));
#11163=CARTESIAN_POINT('Ctrl Pts',(5.80974723471181,0.198712082533353,0.0693141634661021));
#11164=CARTESIAN_POINT('Ctrl Pts',(5.7937414503193,0.182517999394844,0.107475484252794));
#11165=CARTESIAN_POINT('Ctrl Pts',(5.78023922617715,0.166732877511574,0.130251970586776));
#11166=CARTESIAN_POINT('Ctrl Pts',(5.75710894103549,0.130678518444188,0.166306329654162));
#11167=CARTESIAN_POINT('Ctrl Pts',(5.74560158587233,0.107860332287473,0.182341144032028));
#11168=CARTESIAN_POINT('Ctrl Pts',(5.72949374752355,0.0563806217319962,
0.204214038345313));
#11169=CARTESIAN_POINT('Ctrl Pts',(5.725,0.027663639322611,0.21));
#11170=CARTESIAN_POINT('Ctrl Pts',(5.725,6.93889390390723E-18,0.21));
#11171=CARTESIAN_POINT('Ctrl Pts',(5.725,-5.89805981832114E-17,-0.21));
#11172=CARTESIAN_POINT('Ctrl Pts',(5.725,0.0276636393226109,-0.21));
#11173=CARTESIAN_POINT('Ctrl Pts',(5.72949374752355,0.056380621731996,-0.204214038345314));
#11174=CARTESIAN_POINT('Ctrl Pts',(5.74560158587233,0.107860332287473,-0.182341144032028));
#11175=CARTESIAN_POINT('Ctrl Pts',(5.75710894103549,0.130678518444188,-0.166306329654162));
#11176=CARTESIAN_POINT('Ctrl Pts',(5.78023922617715,0.166732877511574,-0.130251970586776));
#11177=CARTESIAN_POINT('Ctrl Pts',(5.7937414503193,0.182517999394844,-0.107475484252795));
#11178=CARTESIAN_POINT('Ctrl Pts',(5.80974723471181,0.198712082533353,-0.0693141634661021));
#11179=CARTESIAN_POINT('Ctrl Pts',(5.81433611385285,0.202908887997328,-0.0559106681449082));
#11180=CARTESIAN_POINT('Ctrl Pts',(5.82070090566933,0.208554382393535,-0.0283388251429182));
#11181=CARTESIAN_POINT('Ctrl Pts',(5.82244719095435,0.21,-0.0141630178371274));
#11182=CARTESIAN_POINT('Ctrl Pts',(5.82244719095435,0.21,-6.24500451351651E-17));
#11183=CARTESIAN_POINT('',(6.17755280904565,0.21,3.29597460435593E-17));
#11184=CARTESIAN_POINT('',(6.275,4.48844336872086E-18,0.21));
#11185=CARTESIAN_POINT('Ctrl Pts',(6.17755280904565,0.21,3.29597460435593E-17));
#11186=CARTESIAN_POINT('Ctrl Pts',(6.17755280904565,0.21,-0.0141630178371274));
#11187=CARTESIAN_POINT('Ctrl Pts',(6.17929909433067,0.208554382393535,-0.0283388251429182));
#11188=CARTESIAN_POINT('Ctrl Pts',(6.18566388614715,0.202908887997328,-0.0559106681449083));
#11189=CARTESIAN_POINT('Ctrl Pts',(6.19025276528819,0.198712082533353,-0.0693141634661022));
#11190=CARTESIAN_POINT('Ctrl Pts',(6.2062585496807,0.182517999394844,-0.107475484252795));
#11191=CARTESIAN_POINT('Ctrl Pts',(6.21976077382285,0.166732877511574,-0.130251970586776));
#11192=CARTESIAN_POINT('Ctrl Pts',(6.24289105896451,0.130678518444188,-0.166306329654162));
#11193=CARTESIAN_POINT('Ctrl Pts',(6.25439841412767,0.107860332287473,-0.182341144032028));
#11194=CARTESIAN_POINT('Ctrl Pts',(6.27050625247645,0.056380621731996,-0.204214038345313));
#11195=CARTESIAN_POINT('Ctrl Pts',(6.275,0.027663639322611,-0.21));
#11196=CARTESIAN_POINT('Ctrl Pts',(6.275,-0.027663639322611,-0.21));
#11197=CARTESIAN_POINT('Ctrl Pts',(6.27050625247645,-0.0563806217319961,
-0.204214038345313));
#11198=CARTESIAN_POINT('Ctrl Pts',(6.25439841412767,-0.107860332287473,
-0.182341144032028));
#11199=CARTESIAN_POINT('Ctrl Pts',(6.24289105896451,-0.130678518444188,
-0.166306329654162));
#11200=CARTESIAN_POINT('Ctrl Pts',(6.21976077382285,-0.166732877511574,
-0.130251970586776));
#11201=CARTESIAN_POINT('Ctrl Pts',(6.2062585496807,-0.182517999394844,-0.107475484252795));
#11202=CARTESIAN_POINT('Ctrl Pts',(6.19025276528819,-0.198712082533353,
-0.0693141634661022));
#11203=CARTESIAN_POINT('Ctrl Pts',(6.18566388614715,-0.202908887997328,
-0.0559106681449083));
#11204=CARTESIAN_POINT('Ctrl Pts',(6.17929909433067,-0.208554382393535,
-0.0283388251429182));
#11205=CARTESIAN_POINT('Ctrl Pts',(6.17755280904565,-0.21,-0.0141630178371274));
#11206=CARTESIAN_POINT('Ctrl Pts',(6.17755280904565,-0.21,0.0141630178371274));
#11207=CARTESIAN_POINT('Ctrl Pts',(6.17929909433067,-0.208554382393535,
0.0283388251429182));
#11208=CARTESIAN_POINT('Ctrl Pts',(6.18566388614715,-0.202908887997328,
0.0559106681449083));
#11209=CARTESIAN_POINT('Ctrl Pts',(6.19025276528819,-0.198712082533353,
0.0693141634661022));
#11210=CARTESIAN_POINT('Ctrl Pts',(6.2062585496807,-0.182517999394844,0.107475484252794));
#11211=CARTESIAN_POINT('Ctrl Pts',(6.21976077382285,-0.166732877511574,
0.130251970586776));
#11212=CARTESIAN_POINT('Ctrl Pts',(6.24289105896451,-0.130678518444188,
0.166306329654162));
#11213=CARTESIAN_POINT('Ctrl Pts',(6.25439841412767,-0.107860332287473,
0.182341144032028));
#11214=CARTESIAN_POINT('Ctrl Pts',(6.27050625247645,-0.0563806217319961,
0.204214038345313));
#11215=CARTESIAN_POINT('Ctrl Pts',(6.275,-0.0276636393226109,0.21));
#11216=CARTESIAN_POINT('Ctrl Pts',(6.275,6.24500451351651E-17,0.21));
#11217=CARTESIAN_POINT('Ctrl Pts',(6.275,3.46944695195361E-17,0.21));
#11218=CARTESIAN_POINT('Ctrl Pts',(6.275,0.027663639322611,0.21));
#11219=CARTESIAN_POINT('Ctrl Pts',(6.27050625247645,0.0563806217319961,
0.204214038345313));
#11220=CARTESIAN_POINT('Ctrl Pts',(6.25439841412767,0.107860332287473,0.182341144032028));
#11221=CARTESIAN_POINT('Ctrl Pts',(6.24289105896451,0.130678518444188,0.166306329654162));
#11222=CARTESIAN_POINT('Ctrl Pts',(6.21976077382285,0.166732877511574,0.130251970586776));
#11223=CARTESIAN_POINT('Ctrl Pts',(6.2062585496807,0.182517999394844,0.107475484252794));
#11224=CARTESIAN_POINT('Ctrl Pts',(6.19025276528819,0.198712082533353,0.0693141634661021));
#11225=CARTESIAN_POINT('Ctrl Pts',(6.18566388614715,0.202908887997328,0.0559106681449083));
#11226=CARTESIAN_POINT('Ctrl Pts',(6.17929909433067,0.208554382393535,0.0283388251429182));
#11227=CARTESIAN_POINT('Ctrl Pts',(6.17755280904565,0.21,0.0141630178371273));
#11228=CARTESIAN_POINT('Ctrl Pts',(6.17755280904565,0.21,-2.77555756156289E-17));
#11229=CARTESIAN_POINT('Origin',(-0.1,0.,0.));
#11230=CARTESIAN_POINT('',(0.,-2.57175827820944E-17,0.21));
#11231=CARTESIAN_POINT('Origin',(0.,0.,0.));
#11232=CARTESIAN_POINT('',(-0.1,-2.57175827820944E-17,0.21));
#11233=CARTESIAN_POINT('Origin',(-0.1,0.82,-0.3));
#11234=CARTESIAN_POINT('',(0.,0.82,-0.3));
#11235=CARTESIAN_POINT('',(0.,1.,-0.3));
#11236=CARTESIAN_POINT('',(0.,0.41,-0.3));
#11237=CARTESIAN_POINT('',(40.,0.82,-0.3));
#11238=CARTESIAN_POINT('',(-0.1,0.82,-0.3));
#11239=CARTESIAN_POINT('',(40.,1.,-0.3));
#11240=CARTESIAN_POINT('',(40.,0.41,-0.3));
#11241=CARTESIAN_POINT('',(-0.05,1.,-0.3));
#11242=CARTESIAN_POINT('Origin',(-0.1,0.82,-0.55));
#11243=CARTESIAN_POINT('',(0.,0.82,-0.55));
#11244=CARTESIAN_POINT('',(0.,0.82,-0.275));
#11245=CARTESIAN_POINT('',(40.,0.82,-0.55));
#11246=CARTESIAN_POINT('',(-0.1,0.82,-0.55));
#11247=CARTESIAN_POINT('',(40.,0.82,-0.275));
#11248=CARTESIAN_POINT('Origin',(-0.1,0.67,-0.55));
#11249=CARTESIAN_POINT('',(0.,0.67,-0.55));
#11250=CARTESIAN_POINT('',(0.,0.335,-0.55));
#11251=CARTESIAN_POINT('',(40.,0.67,-0.55));
#11252=CARTESIAN_POINT('',(-0.1,0.67,-0.55));
#11253=CARTESIAN_POINT('',(40.,0.335,-0.55));
#11254=CARTESIAN_POINT('Origin',(-0.1,0.42,-0.3));
#11255=CARTESIAN_POINT('',(0.,0.42,-0.3));
#11256=CARTESIAN_POINT('',(0.,0.24,-0.12));
#11257=CARTESIAN_POINT('',(40.,0.42,-0.3));
#11258=CARTESIAN_POINT('',(-0.1,0.42,-0.3));
#11259=CARTESIAN_POINT('',(40.,0.24,-0.12));
#11260=CARTESIAN_POINT('Origin',(-0.1,0.42,0.3));
#11261=CARTESIAN_POINT('',(0.,0.42,0.3));
#11262=CARTESIAN_POINT('',(0.,0.42,0.15));
#11263=CARTESIAN_POINT('',(40.,0.42,0.3));
#11264=CARTESIAN_POINT('',(-0.1,0.42,0.3));
#11265=CARTESIAN_POINT('',(40.,0.42,0.15));
#11266=CARTESIAN_POINT('Origin',(-0.1,0.67,0.55));
#11267=CARTESIAN_POINT('',(0.,0.67,0.55));
#11268=CARTESIAN_POINT('',(6.93889390390723E-18,0.365,0.245));
#11269=CARTESIAN_POINT('',(40.,0.67,0.55));
#11270=CARTESIAN_POINT('',(-0.1,0.67,0.55));
#11271=CARTESIAN_POINT('',(40.,0.365,0.245));
#11272=CARTESIAN_POINT('Origin',(-0.1,0.82,0.55));
#11273=CARTESIAN_POINT('',(0.,0.82,0.55));
#11274=CARTESIAN_POINT('',(0.,0.41,0.55));
#11275=CARTESIAN_POINT('',(40.,0.82,0.55));
#11276=CARTESIAN_POINT('',(-0.1,0.82,0.55));
#11277=CARTESIAN_POINT('',(40.,0.41,0.55));
#11278=CARTESIAN_POINT('Origin',(-0.1,0.82,0.3));
#11279=CARTESIAN_POINT('',(0.,0.82,0.3));
#11280=CARTESIAN_POINT('',(0.,0.82,0.15));
#11281=CARTESIAN_POINT('',(40.,0.82,0.3));
#11282=CARTESIAN_POINT('',(-0.1,0.82,0.3));
#11283=CARTESIAN_POINT('',(40.,0.82,0.15));
#11284=CARTESIAN_POINT('Origin',(-0.1,1.05,0.3));
#11285=CARTESIAN_POINT('',(0.,1.,0.3));
#11286=CARTESIAN_POINT('',(0.,0.525,0.3));
#11287=CARTESIAN_POINT('',(40.,1.,0.3));
#11288=CARTESIAN_POINT('',(-0.05,1.,0.3));
#11289=CARTESIAN_POINT('',(40.,0.525,0.3));
#11290=CARTESIAN_POINT('Origin',(-0.1,-0.3,-0.82));
#11291=CARTESIAN_POINT('',(0.,-0.3,-0.82));
#11292=CARTESIAN_POINT('',(0.,-0.3,-1.));
#11293=CARTESIAN_POINT('',(0.,-0.3,-0.41));
#11294=CARTESIAN_POINT('',(40.,-0.3,-0.82));
#11295=CARTESIAN_POINT('',(-0.1,-0.3,-0.82));
#11296=CARTESIAN_POINT('',(40.,-0.3,-1.));
#11297=CARTESIAN_POINT('',(40.,-0.3,-0.41));
#11298=CARTESIAN_POINT('',(-0.05,-0.3,-1.));
#11299=CARTESIAN_POINT('Origin',(-0.1,-0.55,-0.82));
#11300=CARTESIAN_POINT('',(0.,-0.55,-0.82));
#11301=CARTESIAN_POINT('',(0.,-0.275,-0.82));
#11302=CARTESIAN_POINT('',(40.,-0.55,-0.82));
#11303=CARTESIAN_POINT('',(-0.1,-0.55,-0.82));
#11304=CARTESIAN_POINT('',(40.,-0.275,-0.82));
#11305=CARTESIAN_POINT('Origin',(-0.1,-0.55,-0.67));
#11306=CARTESIAN_POINT('',(0.,-0.55,-0.67));
#11307=CARTESIAN_POINT('',(0.,-0.55,-0.335));
#11308=CARTESIAN_POINT('',(40.,-0.55,-0.67));
#11309=CARTESIAN_POINT('',(-0.1,-0.55,-0.67));
#11310=CARTESIAN_POINT('',(40.,-0.55,-0.335));
#11311=CARTESIAN_POINT('Origin',(-0.1,-0.3,-0.42));
#11312=CARTESIAN_POINT('',(0.,-0.3,-0.42));
#11313=CARTESIAN_POINT('',(0.,-0.12,-0.24));
#11314=CARTESIAN_POINT('',(40.,-0.3,-0.42));
#11315=CARTESIAN_POINT('',(-0.1,-0.3,-0.42));
#11316=CARTESIAN_POINT('',(40.,-0.12,-0.24));
#11317=CARTESIAN_POINT('Origin',(-0.1,0.3,-0.42));
#11318=CARTESIAN_POINT('',(0.,0.3,-0.42));
#11319=CARTESIAN_POINT('',(0.,0.15,-0.42));
#11320=CARTESIAN_POINT('',(40.,0.3,-0.42));
#11321=CARTESIAN_POINT('',(-0.1,0.3,-0.42));
#11322=CARTESIAN_POINT('',(40.,0.15,-0.42));
#11323=CARTESIAN_POINT('Origin',(-0.1,0.55,-0.67));
#11324=CARTESIAN_POINT('',(0.,0.55,-0.67));
#11325=CARTESIAN_POINT('',(0.,0.245,-0.365));
#11326=CARTESIAN_POINT('',(40.,0.55,-0.67));
#11327=CARTESIAN_POINT('',(-0.1,0.55,-0.67));
#11328=CARTESIAN_POINT('',(40.,0.245,-0.365));
#11329=CARTESIAN_POINT('Origin',(-0.1,0.55,-0.82));
#11330=CARTESIAN_POINT('',(0.,0.55,-0.82));
#11331=CARTESIAN_POINT('',(0.,0.55,-0.41));
#11332=CARTESIAN_POINT('',(40.,0.55,-0.82));
#11333=CARTESIAN_POINT('',(-0.1,0.55,-0.82));
#11334=CARTESIAN_POINT('',(40.,0.55,-0.41));
#11335=CARTESIAN_POINT('Origin',(-0.1,0.3,-0.82));
#11336=CARTESIAN_POINT('',(0.,0.3,-0.82));
#11337=CARTESIAN_POINT('',(0.,0.15,-0.82));
#11338=CARTESIAN_POINT('',(40.,0.3,-0.82));
#11339=CARTESIAN_POINT('',(-0.1,0.3,-0.82));
#11340=CARTESIAN_POINT('',(40.,0.15,-0.82));
#11341=CARTESIAN_POINT('Origin',(-0.1,0.3,-1.05));
#11342=CARTESIAN_POINT('',(0.,0.3,-1.));
#11343=CARTESIAN_POINT('',(0.,0.3,-0.525));
#11344=CARTESIAN_POINT('',(40.,0.3,-1.));
#11345=CARTESIAN_POINT('',(-0.05,0.3,-1.));
#11346=CARTESIAN_POINT('',(40.,0.3,-0.525));
#11347=CARTESIAN_POINT('Origin',(-0.1,-0.82,0.3));
#11348=CARTESIAN_POINT('',(0.,-0.82,0.3));
#11349=CARTESIAN_POINT('',(0.,-1.,0.3));
#11350=CARTESIAN_POINT('',(0.,-0.41,0.3));
#11351=CARTESIAN_POINT('',(40.,-0.82,0.3));
#11352=CARTESIAN_POINT('',(-0.1,-0.82,0.3));
#11353=CARTESIAN_POINT('',(40.,-1.,0.3));
#11354=CARTESIAN_POINT('',(40.,-0.41,0.3));
#11355=CARTESIAN_POINT('',(-0.05,-1.,0.3));
#11356=CARTESIAN_POINT('Origin',(-0.1,-0.82,0.55));
#11357=CARTESIAN_POINT('',(0.,-0.82,0.55));
#11358=CARTESIAN_POINT('',(0.,-0.82,0.275));
#11359=CARTESIAN_POINT('',(40.,-0.82,0.55));
#11360=CARTESIAN_POINT('',(-0.1,-0.82,0.55));
#11361=CARTESIAN_POINT('',(40.,-0.82,0.275));
#11362=CARTESIAN_POINT('Origin',(-0.1,-0.67,0.55));
#11363=CARTESIAN_POINT('',(0.,-0.67,0.55));
#11364=CARTESIAN_POINT('',(0.,-0.335,0.55));
#11365=CARTESIAN_POINT('',(40.,-0.67,0.55));
#11366=CARTESIAN_POINT('',(-0.1,-0.67,0.55));
#11367=CARTESIAN_POINT('',(40.,-0.335,0.55));
#11368=CARTESIAN_POINT('Origin',(-0.1,-0.42,0.3));
#11369=CARTESIAN_POINT('',(0.,-0.42,0.3));
#11370=CARTESIAN_POINT('',(-6.93889390390723E-18,-0.24,0.12));
#11371=CARTESIAN_POINT('',(40.,-0.42,0.3));
#11372=CARTESIAN_POINT('',(-0.1,-0.42,0.3));
#11373=CARTESIAN_POINT('',(40.,-0.24,0.12));
#11374=CARTESIAN_POINT('Origin',(-0.1,-0.42,-0.3));
#11375=CARTESIAN_POINT('',(0.,-0.42,-0.3));
#11376=CARTESIAN_POINT('',(0.,-0.42,-0.15));
#11377=CARTESIAN_POINT('',(40.,-0.42,-0.3));
#11378=CARTESIAN_POINT('',(-0.1,-0.42,-0.3));
#11379=CARTESIAN_POINT('',(40.,-0.42,-0.15));
#11380=CARTESIAN_POINT('Origin',(-0.1,-0.67,-0.55));
#11381=CARTESIAN_POINT('',(0.,-0.67,-0.55));
#11382=CARTESIAN_POINT('',(0.,-0.365,-0.245));
#11383=CARTESIAN_POINT('',(40.,-0.67,-0.55));
#11384=CARTESIAN_POINT('',(-0.1,-0.67,-0.55));
#11385=CARTESIAN_POINT('',(40.,-0.365,-0.245));
#11386=CARTESIAN_POINT('Origin',(-0.1,-0.82,-0.55));
#11387=CARTESIAN_POINT('',(0.,-0.82,-0.55));
#11388=CARTESIAN_POINT('',(0.,-0.41,-0.55));
#11389=CARTESIAN_POINT('',(40.,-0.82,-0.55));
#11390=CARTESIAN_POINT('',(-0.1,-0.82,-0.55));
#11391=CARTESIAN_POINT('',(40.,-0.41,-0.55));
#11392=CARTESIAN_POINT('Origin',(-0.1,-0.82,-0.3));
#11393=CARTESIAN_POINT('',(0.,-0.82,-0.3));
#11394=CARTESIAN_POINT('',(0.,-0.82,-0.15));
#11395=CARTESIAN_POINT('',(40.,-0.82,-0.3));
#11396=CARTESIAN_POINT('',(-0.1,-0.82,-0.3));
#11397=CARTESIAN_POINT('',(40.,-0.82,-0.15));
#11398=CARTESIAN_POINT('Origin',(-0.1,-1.05,-0.3));
#11399=CARTESIAN_POINT('',(0.,-1.,-0.3));
#11400=CARTESIAN_POINT('',(0.,-0.525,-0.3));
#11401=CARTESIAN_POINT('',(40.,-1.,-0.3));
#11402=CARTESIAN_POINT('',(-0.05,-1.,-0.3));
#11403=CARTESIAN_POINT('',(40.,-0.525,-0.3));
#11404=CARTESIAN_POINT('Origin',(-0.1,0.3,0.82));
#11405=CARTESIAN_POINT('',(0.,0.3,0.82));
#11406=CARTESIAN_POINT('',(0.,0.3,1.));
#11407=CARTESIAN_POINT('',(0.,0.3,0.41));
#11408=CARTESIAN_POINT('',(40.,0.3,0.82));
#11409=CARTESIAN_POINT('',(-0.1,0.3,0.82));
#11410=CARTESIAN_POINT('',(40.,0.3,1.));
#11411=CARTESIAN_POINT('',(40.,0.3,0.41));
#11412=CARTESIAN_POINT('',(-0.05,0.3,1.));
#11413=CARTESIAN_POINT('Origin',(-0.1,0.55,0.82));
#11414=CARTESIAN_POINT('',(0.,0.55,0.82));
#11415=CARTESIAN_POINT('',(0.,0.275,0.82));
#11416=CARTESIAN_POINT('',(40.,0.55,0.82));
#11417=CARTESIAN_POINT('',(-0.1,0.55,0.82));
#11418=CARTESIAN_POINT('',(40.,0.275,0.82));
#11419=CARTESIAN_POINT('Origin',(-0.1,0.55,0.67));
#11420=CARTESIAN_POINT('',(0.,0.55,0.67));
#11421=CARTESIAN_POINT('',(0.,0.55,0.335));
#11422=CARTESIAN_POINT('',(40.,0.55,0.67));
#11423=CARTESIAN_POINT('',(-0.1,0.55,0.67));
#11424=CARTESIAN_POINT('',(40.,0.55,0.335));
#11425=CARTESIAN_POINT('Origin',(-0.1,0.3,0.42));
#11426=CARTESIAN_POINT('',(0.,0.3,0.42));
#11427=CARTESIAN_POINT('',(6.93889390390723E-18,0.12,0.24));
#11428=CARTESIAN_POINT('',(40.,0.3,0.42));
#11429=CARTESIAN_POINT('',(-0.1,0.3,0.42));
#11430=CARTESIAN_POINT('',(40.,0.12,0.24));
#11431=CARTESIAN_POINT('Origin',(-0.1,-0.3,0.42));
#11432=CARTESIAN_POINT('',(0.,-0.3,0.42));
#11433=CARTESIAN_POINT('',(0.,-0.15,0.42));
#11434=CARTESIAN_POINT('',(40.,-0.3,0.42));
#11435=CARTESIAN_POINT('',(-0.1,-0.3,0.42));
#11436=CARTESIAN_POINT('',(40.,-0.15,0.42));
#11437=CARTESIAN_POINT('Origin',(-0.1,-0.55,0.67));
#11438=CARTESIAN_POINT('',(0.,-0.55,0.67));
#11439=CARTESIAN_POINT('',(6.93889390390723E-18,-0.245,0.365));
#11440=CARTESIAN_POINT('',(40.,-0.55,0.67));
#11441=CARTESIAN_POINT('',(-0.1,-0.55,0.67));
#11442=CARTESIAN_POINT('',(40.,-0.245,0.365));
#11443=CARTESIAN_POINT('Origin',(-0.1,-0.55,0.82));
#11444=CARTESIAN_POINT('',(0.,-0.55,0.82));
#11445=CARTESIAN_POINT('',(0.,-0.55,0.41));
#11446=CARTESIAN_POINT('',(40.,-0.55,0.82));
#11447=CARTESIAN_POINT('',(-0.1,-0.55,0.82));
#11448=CARTESIAN_POINT('',(40.,-0.55,0.41));
#11449=CARTESIAN_POINT('Origin',(-0.1,-0.3,0.82));
#11450=CARTESIAN_POINT('',(0.,-0.3,0.82));
#11451=CARTESIAN_POINT('',(0.,-0.15,0.82));
#11452=CARTESIAN_POINT('',(40.,-0.3,0.82));
#11453=CARTESIAN_POINT('',(-0.1,-0.3,0.82));
#11454=CARTESIAN_POINT('',(40.,-0.15,0.82));
#11455=CARTESIAN_POINT('Origin',(-0.1,-0.3,1.05));
#11456=CARTESIAN_POINT('',(0.,-0.3,1.));
#11457=CARTESIAN_POINT('',(0.,-0.3,0.525));
#11458=CARTESIAN_POINT('',(40.,-0.3,1.));
#11459=CARTESIAN_POINT('',(-0.05,-0.3,1.));
#11460=CARTESIAN_POINT('',(40.,-0.3,0.525));
#11461=CARTESIAN_POINT('Origin',(-0.1,0.,0.));
#11462=CARTESIAN_POINT('',(40.,2.57175827820944E-17,0.21));
#11463=CARTESIAN_POINT('',(-0.1,-2.57175827820944E-17,0.21));
#11464=CARTESIAN_POINT('Origin',(40.,0.,0.));
#11465=CARTESIAN_POINT('Origin',(0.,1.,-1.));
#11466=CARTESIAN_POINT('',(0.,1.,1.));
#11467=CARTESIAN_POINT('',(0.,1.,-1.));
#11468=CARTESIAN_POINT('',(40.,1.,1.));
#11469=CARTESIAN_POINT('',(0.,1.,1.));
#11470=CARTESIAN_POINT('',(40.,1.,-1.));
#11471=CARTESIAN_POINT('Origin',(0.,1.,-1.));
#11472=CARTESIAN_POINT('',(40.,1.,-1.));
#11473=CARTESIAN_POINT('',(40.,1.,-1.));
#11474=CARTESIAN_POINT('',(0.,1.,-1.));
#11475=CARTESIAN_POINT('',(0.,1.,-1.));
#11476=CARTESIAN_POINT('',(0.,1.,-1.));
#11477=CARTESIAN_POINT('Origin',(0.,-1.,-1.));
#11478=CARTESIAN_POINT('',(0.,-1.,-1.));
#11479=CARTESIAN_POINT('',(40.,-1.,-1.));
#11480=CARTESIAN_POINT('Origin',(0.,-1.,-1.));
#11481=CARTESIAN_POINT('',(40.,-1.,-1.));
#11482=CARTESIAN_POINT('',(40.,-1.,-1.));
#11483=CARTESIAN_POINT('',(0.,-1.,-1.));
#11484=CARTESIAN_POINT('',(0.,-1.,-1.));
#11485=CARTESIAN_POINT('',(0.,-1.,-1.));
#11486=CARTESIAN_POINT('Origin',(0.,-1.,1.));
#11487=CARTESIAN_POINT('',(0.,-1.,1.));
#11488=CARTESIAN_POINT('',(40.,-1.,1.));
#11489=CARTESIAN_POINT('Origin',(0.,-1.,1.));
#11490=CARTESIAN_POINT('',(40.,-1.,1.));
#11491=CARTESIAN_POINT('',(40.,-1.,1.));
#11492=CARTESIAN_POINT('',(0.,-1.,1.));
#11493=CARTESIAN_POINT('',(0.,-1.,1.));
#11494=CARTESIAN_POINT('',(0.,-1.,1.));
#11495=CARTESIAN_POINT('Origin',(0.,1.,1.));
#11496=CARTESIAN_POINT('',(0.,1.,1.));
#11497=CARTESIAN_POINT('',(40.,1.,1.));
#11498=CARTESIAN_POINT('Origin',(0.,1.,1.));
#11499=CARTESIAN_POINT('',(40.,1.,1.));
#11500=CARTESIAN_POINT('',(0.,1.,1.));
#11501=CARTESIAN_POINT('Origin',(40.,0.,0.));
#11502=CARTESIAN_POINT('Origin',(0.,0.,0.));
#13747=UNCERTAINTY_MEASURE_WITH_UNIT(LENGTH_MEASURE(0.001),#13822,
'DISTANCE_ACCURACY_VALUE',
'Maximum model space distance between geometric entities at asserted c
onnectivities');
#13782=UNCERTAINTY_MEASURE_WITH_UNIT(LENGTH_MEASURE(0.001),#13822,
'DISTANCE_ACCURACY_VALUE',
'Maximum model space distance between geometric entities at asserted c
onnectivities');
#13786=(
GEOMETRIC_REPRESENTATION_CONTEXT(3)
GLOBAL_UNCERTAINTY_ASSIGNED_CONTEXT((#13747))
GLOBAL_UNIT_ASSIGNED_CONTEXT((#13822,#13824,#13825))
REPRESENTATION_CONTEXT('','3D')
);
#13821=(
GEOMETRIC_REPRESENTATION_CONTEXT(3)
GLOBAL_UNCERTAINTY_ASSIGNED_CONTEXT((#13782))
GLOBAL_UNIT_ASSIGNED_CONTEXT((#13822,#13824,#13825))
REPRESENTATION_CONTEXT('','3D')
);
#13822=(
LENGTH_UNIT()
NAMED_UNIT(*)
SI_UNIT(.CENTI.,.METRE.)
);
#13824=(
NAMED_UNIT(*)
PLANE_ANGLE_UNIT()
SI_UNIT($,.RADIAN.)
);
#13825=(
NAMED_UNIT(*)
SI_UNIT($,.STERADIAN.)
SOLID_ANGLE_UNIT()
);
#13829=SHAPE_DEFINITION_REPRESENTATION(#13867,#13999);
#13867=PRODUCT_DEFINITION_SHAPE('',$,#14038);
#13999=SHAPE_REPRESENTATION('',(#8069),#13786);
#14034=PRODUCT_DEFINITION_CONTEXT('part definition',#14150,'design');
#14038=PRODUCT_DEFINITION('Drilled 400 mm rail','Drilled 400 mm rail',#14076,
#14034);
#14076=PRODUCT_DEFINITION_FORMATION('',$,#14155);
#14150=APPLICATION_CONTEXT(
'Core Data for Automotive Mechanical Design Process');
#14151=PRODUCT_CONTEXT('part definition',#14150,'mechanical');
#14155=PRODUCT('Drilled 400 mm rail','Drilled 400 mm rail',
'Drilled 400 mm rail',(#14151));
#14191=PRESENTATION_STYLE_ASSIGNMENT((#14196));
#14196=SURFACE_STYLE_USAGE(.BOTH.,#14201);
#14201=SURFACE_SIDE_STYLE('',(#14206));
#14206=SURFACE_STYLE_FILL_AREA(#14211);
#14211=FILL_AREA_STYLE('CAD Library Painted - Steel gray',(#14216));
#14216=FILL_AREA_STYLE_COLOUR('CAD Library Painted - Steel gray',#14221);
#14221=COLOUR_RGB('CAD Library Painted - Steel gray',0.592156862745098,
0.631372549019608,0.67843137254902);
ENDSEC;
END-ISO-10303-21;
